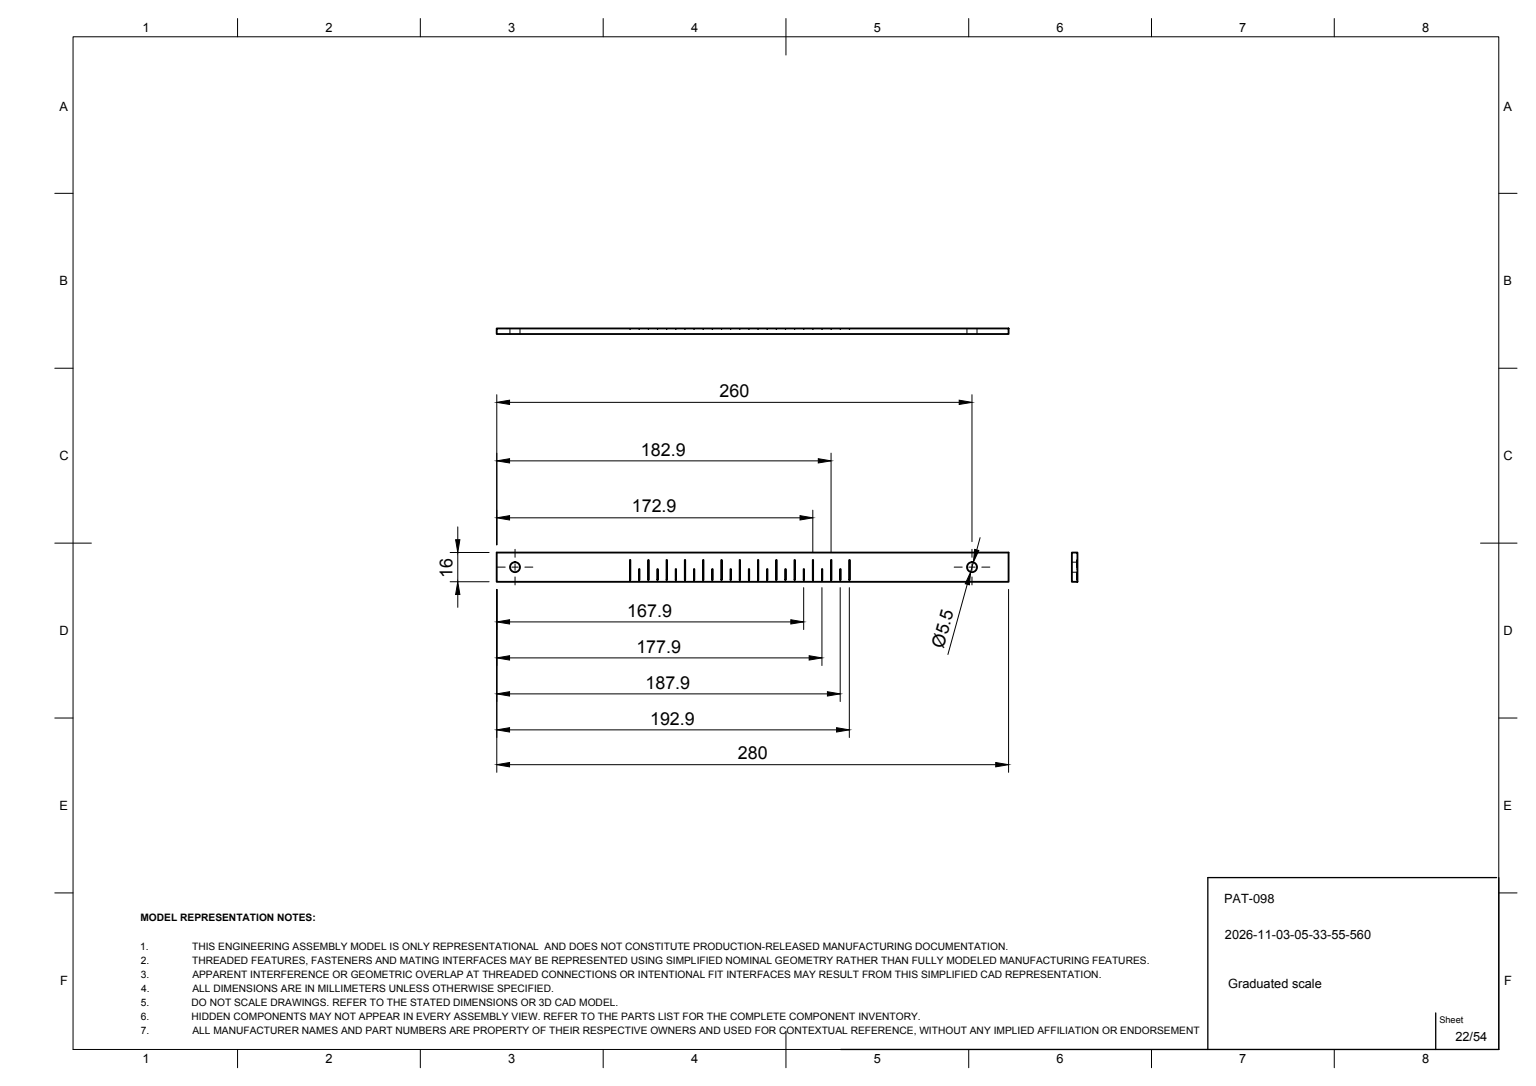
ISO-10303-21;
HEADER;
/* Generated by software containing ST-Developer
 * from STEP Tools, Inc. (www.steptools.com) 
 */

FILE_DESCRIPTION(
/* description */ ('Spring compression tester'),
/* implementation_level */ '2;1');

FILE_NAME(
/* name */ 'Graduated scale.step',
/* time_stamp */ '2026-10-28T03:24:11-07:00',
/* author */ (''),
/* organization */ (''),
/* preprocessor_version */ 'ST-DEVELOPER v20.2',
/* originating_system */ 'Autodesk Translation Framework v15.17.0.0',
/* authorisation */ '');

FILE_SCHEMA (('AUTOMOTIVE_DESIGN { 1 0 10303 214 3 1 1 }'));
ENDSEC;

DATA;
#10=MECHANICAL_DESIGN_GEOMETRIC_PRESENTATION_REPRESENTATION('',(#1123),#43521);
#1003=SHAPE_REPRESENTATION_RELATIONSHIP('SRR','None',#43815,#1063);
#1063=ADVANCED_BREP_SHAPE_REPRESENTATION('',(#1198),#43475);
#1123=STYLED_ITEM('',(#44216),#1198);
#1198=MANIFOLD_SOLID_BREP('Body1',#18560);
#1410=FACE_BOUND('',#3758,.T.);
#1411=FACE_BOUND('',#3759,.T.);
#1412=FACE_BOUND('',#3762,.T.);
#1413=FACE_BOUND('',#3763,.T.);
#1414=FACE_BOUND('',#3764,.T.);
#1415=FACE_BOUND('',#3765,.T.);
#1416=FACE_BOUND('',#3766,.T.);
#1417=FACE_BOUND('',#3767,.T.);
#1418=FACE_BOUND('',#3768,.T.);
#1419=FACE_BOUND('',#3769,.T.);
#1420=FACE_BOUND('',#3770,.T.);
#1421=FACE_BOUND('',#3771,.T.);
#1422=FACE_BOUND('',#3772,.T.);
#1423=FACE_BOUND('',#3773,.T.);
#1424=FACE_BOUND('',#3774,.T.);
#1425=FACE_BOUND('',#3775,.T.);
#1426=FACE_BOUND('',#3776,.T.);
#1427=FACE_BOUND('',#3777,.T.);
#1428=FACE_BOUND('',#3778,.T.);
#1429=FACE_BOUND('',#3779,.T.);
#1430=FACE_BOUND('',#3780,.T.);
#1431=FACE_BOUND('',#3781,.T.);
#1432=FACE_BOUND('',#3782,.T.);
#1433=FACE_BOUND('',#3783,.T.);
#1434=FACE_BOUND('',#3784,.T.);
#1435=FACE_BOUND('',#3785,.T.);
#1436=FACE_BOUND('',#3786,.T.);
#1437=FACE_BOUND('',#3787,.T.);
#1438=FACE_BOUND('',#3788,.T.);
#1728=PLANE('',#19783);
#1729=PLANE('',#19784);
#1730=PLANE('',#19785);
#1731=PLANE('',#19786);
#1732=PLANE('',#19787);
#1733=PLANE('',#19788);
#1734=PLANE('',#19789);
#1735=PLANE('',#19790);
#1736=PLANE('',#19791);
#1737=PLANE('',#19792);
#1738=PLANE('',#19793);
#1739=PLANE('',#19794);
#1740=PLANE('',#19795);
#1741=PLANE('',#19796);
#1742=PLANE('',#19797);
#1743=PLANE('',#19798);
#1744=PLANE('',#19799);
#1745=PLANE('',#19800);
#1746=PLANE('',#19801);
#1747=PLANE('',#19802);
#1748=PLANE('',#19803);
#1749=PLANE('',#19804);
#1750=PLANE('',#19805);
#1751=PLANE('',#19806);
#1752=PLANE('',#19807);
#1753=PLANE('',#19808);
#1754=PLANE('',#19809);
#1755=PLANE('',#19810);
#1756=PLANE('',#19811);
#1757=PLANE('',#19812);
#1758=PLANE('',#19813);
#1759=PLANE('',#19814);
#1760=PLANE('',#19815);
#1761=PLANE('',#19816);
#1762=PLANE('',#19817);
#1763=PLANE('',#19818);
#1764=PLANE('',#19819);
#1765=PLANE('',#19820);
#1766=PLANE('',#19821);
#1767=PLANE('',#19822);
#1768=PLANE('',#19823);
#1769=PLANE('',#19824);
#1770=PLANE('',#19825);
#1771=PLANE('',#19826);
#1772=PLANE('',#19827);
#1773=PLANE('',#19828);
#1774=PLANE('',#19829);
#1775=PLANE('',#19830);
#1776=PLANE('',#19831);
#1777=PLANE('',#19832);
#1778=PLANE('',#19833);
#1779=PLANE('',#19834);
#1780=PLANE('',#19835);
#1781=PLANE('',#19836);
#1782=PLANE('',#19837);
#1783=PLANE('',#19838);
#1784=PLANE('',#19839);
#1785=PLANE('',#19840);
#1786=PLANE('',#19841);
#1787=PLANE('',#19842);
#1788=PLANE('',#19843);
#1789=PLANE('',#19844);
#1790=PLANE('',#19845);
#1791=PLANE('',#19846);
#1792=PLANE('',#19847);
#1793=PLANE('',#19848);
#1794=PLANE('',#19849);
#1795=PLANE('',#19850);
#1796=PLANE('',#19851);
#1797=PLANE('',#19852);
#1798=PLANE('',#19853);
#1799=PLANE('',#19854);
#1800=PLANE('',#19855);
#1801=PLANE('',#19856);
#1802=PLANE('',#19857);
#1803=PLANE('',#19858);
#1804=PLANE('',#19859);
#1805=PLANE('',#19860);
#1806=PLANE('',#19861);
#1807=PLANE('',#19862);
#1808=PLANE('',#19863);
#1809=PLANE('',#19864);
#1810=PLANE('',#19865);
#1811=PLANE('',#19866);
#1812=PLANE('',#19867);
#1813=PLANE('',#19868);
#1814=PLANE('',#19869);
#1815=PLANE('',#19870);
#1816=PLANE('',#19871);
#1817=PLANE('',#19872);
#1818=PLANE('',#19873);
#1819=PLANE('',#19874);
#1820=PLANE('',#19875);
#1821=PLANE('',#19876);
#1822=PLANE('',#19877);
#1823=PLANE('',#19878);
#1824=PLANE('',#19879);
#1825=PLANE('',#19880);
#1826=PLANE('',#19881);
#1827=PLANE('',#19882);
#1828=PLANE('',#19883);
#1829=PLANE('',#19884);
#1830=PLANE('',#19885);
#1831=PLANE('',#19886);
#1832=PLANE('',#19887);
#1833=PLANE('',#19888);
#1834=PLANE('',#19889);
#1835=PLANE('',#19890);
#1836=PLANE('',#19891);
#1837=PLANE('',#19892);
#1838=PLANE('',#19893);
#1839=PLANE('',#19894);
#1840=PLANE('',#19895);
#1841=PLANE('',#19896);
#1842=PLANE('',#19897);
#1843=PLANE('',#19898);
#1844=PLANE('',#19899);
#1845=PLANE('',#19900);
#1846=PLANE('',#19901);
#1847=PLANE('',#19902);
#1848=PLANE('',#19903);
#1849=PLANE('',#19904);
#1850=PLANE('',#19905);
#1851=PLANE('',#19906);
#1852=PLANE('',#19907);
#1853=PLANE('',#19914);
#1854=PLANE('',#19915);
#1855=PLANE('',#19916);
#1856=PLANE('',#19917);
#1857=PLANE('',#19918);
#1858=PLANE('',#19919);
#2419=FACE_OUTER_BOUND('',#3629,.T.);
#2420=FACE_OUTER_BOUND('',#3630,.T.);
#2421=FACE_OUTER_BOUND('',#3631,.T.);
#2422=FACE_OUTER_BOUND('',#3632,.T.);
#2423=FACE_OUTER_BOUND('',#3633,.T.);
#2424=FACE_OUTER_BOUND('',#3634,.T.);
#2425=FACE_OUTER_BOUND('',#3635,.T.);
#2426=FACE_OUTER_BOUND('',#3636,.T.);
#2427=FACE_OUTER_BOUND('',#3637,.T.);
#2428=FACE_OUTER_BOUND('',#3638,.T.);
#2429=FACE_OUTER_BOUND('',#3639,.T.);
#2430=FACE_OUTER_BOUND('',#3640,.T.);
#2431=FACE_OUTER_BOUND('',#3641,.T.);
#2432=FACE_OUTER_BOUND('',#3642,.T.);
#2433=FACE_OUTER_BOUND('',#3643,.T.);
#2434=FACE_OUTER_BOUND('',#3644,.T.);
#2435=FACE_OUTER_BOUND('',#3645,.T.);
#2436=FACE_OUTER_BOUND('',#3646,.T.);
#2437=FACE_OUTER_BOUND('',#3647,.T.);
#2438=FACE_OUTER_BOUND('',#3648,.T.);
#2439=FACE_OUTER_BOUND('',#3649,.T.);
#2440=FACE_OUTER_BOUND('',#3650,.T.);
#2441=FACE_OUTER_BOUND('',#3651,.T.);
#2442=FACE_OUTER_BOUND('',#3652,.T.);
#2443=FACE_OUTER_BOUND('',#3653,.T.);
#2444=FACE_OUTER_BOUND('',#3654,.T.);
#2445=FACE_OUTER_BOUND('',#3655,.T.);
#2446=FACE_OUTER_BOUND('',#3656,.T.);
#2447=FACE_OUTER_BOUND('',#3657,.T.);
#2448=FACE_OUTER_BOUND('',#3658,.T.);
#2449=FACE_OUTER_BOUND('',#3659,.T.);
#2450=FACE_OUTER_BOUND('',#3660,.T.);
#2451=FACE_OUTER_BOUND('',#3661,.T.);
#2452=FACE_OUTER_BOUND('',#3662,.T.);
#2453=FACE_OUTER_BOUND('',#3663,.T.);
#2454=FACE_OUTER_BOUND('',#3664,.T.);
#2455=FACE_OUTER_BOUND('',#3665,.T.);
#2456=FACE_OUTER_BOUND('',#3666,.T.);
#2457=FACE_OUTER_BOUND('',#3667,.T.);
#2458=FACE_OUTER_BOUND('',#3668,.T.);
#2459=FACE_OUTER_BOUND('',#3669,.T.);
#2460=FACE_OUTER_BOUND('',#3670,.T.);
#2461=FACE_OUTER_BOUND('',#3671,.T.);
#2462=FACE_OUTER_BOUND('',#3672,.T.);
#2463=FACE_OUTER_BOUND('',#3673,.T.);
#2464=FACE_OUTER_BOUND('',#3674,.T.);
#2465=FACE_OUTER_BOUND('',#3675,.T.);
#2466=FACE_OUTER_BOUND('',#3676,.T.);
#2467=FACE_OUTER_BOUND('',#3677,.T.);
#2468=FACE_OUTER_BOUND('',#3678,.T.);
#2469=FACE_OUTER_BOUND('',#3679,.T.);
#2470=FACE_OUTER_BOUND('',#3680,.T.);
#2471=FACE_OUTER_BOUND('',#3681,.T.);
#2472=FACE_OUTER_BOUND('',#3682,.T.);
#2473=FACE_OUTER_BOUND('',#3683,.T.);
#2474=FACE_OUTER_BOUND('',#3684,.T.);
#2475=FACE_OUTER_BOUND('',#3685,.T.);
#2476=FACE_OUTER_BOUND('',#3686,.T.);
#2477=FACE_OUTER_BOUND('',#3687,.T.);
#2478=FACE_OUTER_BOUND('',#3688,.T.);
#2479=FACE_OUTER_BOUND('',#3689,.T.);
#2480=FACE_OUTER_BOUND('',#3690,.T.);
#2481=FACE_OUTER_BOUND('',#3691,.T.);
#2482=FACE_OUTER_BOUND('',#3692,.T.);
#2483=FACE_OUTER_BOUND('',#3693,.T.);
#2484=FACE_OUTER_BOUND('',#3694,.T.);
#2485=FACE_OUTER_BOUND('',#3695,.T.);
#2486=FACE_OUTER_BOUND('',#3696,.T.);
#2487=FACE_OUTER_BOUND('',#3697,.T.);
#2488=FACE_OUTER_BOUND('',#3698,.T.);
#2489=FACE_OUTER_BOUND('',#3699,.T.);
#2490=FACE_OUTER_BOUND('',#3700,.T.);
#2491=FACE_OUTER_BOUND('',#3701,.T.);
#2492=FACE_OUTER_BOUND('',#3702,.T.);
#2493=FACE_OUTER_BOUND('',#3703,.T.);
#2494=FACE_OUTER_BOUND('',#3704,.T.);
#2495=FACE_OUTER_BOUND('',#3705,.T.);
#2496=FACE_OUTER_BOUND('',#3706,.T.);
#2497=FACE_OUTER_BOUND('',#3707,.T.);
#2498=FACE_OUTER_BOUND('',#3708,.T.);
#2499=FACE_OUTER_BOUND('',#3709,.T.);
#2500=FACE_OUTER_BOUND('',#3710,.T.);
#2501=FACE_OUTER_BOUND('',#3711,.T.);
#2502=FACE_OUTER_BOUND('',#3712,.T.);
#2503=FACE_OUTER_BOUND('',#3713,.T.);
#2504=FACE_OUTER_BOUND('',#3714,.T.);
#2505=FACE_OUTER_BOUND('',#3715,.T.);
#2506=FACE_OUTER_BOUND('',#3716,.T.);
#2507=FACE_OUTER_BOUND('',#3717,.T.);
#2508=FACE_OUTER_BOUND('',#3718,.T.);
#2509=FACE_OUTER_BOUND('',#3719,.T.);
#2510=FACE_OUTER_BOUND('',#3720,.T.);
#2511=FACE_OUTER_BOUND('',#3721,.T.);
#2512=FACE_OUTER_BOUND('',#3722,.T.);
#2513=FACE_OUTER_BOUND('',#3723,.T.);
#2514=FACE_OUTER_BOUND('',#3724,.T.);
#2515=FACE_OUTER_BOUND('',#3725,.T.);
#2516=FACE_OUTER_BOUND('',#3726,.T.);
#2517=FACE_OUTER_BOUND('',#3727,.T.);
#2518=FACE_OUTER_BOUND('',#3728,.T.);
#2519=FACE_OUTER_BOUND('',#3729,.T.);
#2520=FACE_OUTER_BOUND('',#3730,.T.);
#2521=FACE_OUTER_BOUND('',#3731,.T.);
#2522=FACE_OUTER_BOUND('',#3732,.T.);
#2523=FACE_OUTER_BOUND('',#3733,.T.);
#2524=FACE_OUTER_BOUND('',#3734,.T.);
#2525=FACE_OUTER_BOUND('',#3735,.T.);
#2526=FACE_OUTER_BOUND('',#3736,.T.);
#2527=FACE_OUTER_BOUND('',#3737,.T.);
#2528=FACE_OUTER_BOUND('',#3738,.T.);
#2529=FACE_OUTER_BOUND('',#3739,.T.);
#2530=FACE_OUTER_BOUND('',#3740,.T.);
#2531=FACE_OUTER_BOUND('',#3741,.T.);
#2532=FACE_OUTER_BOUND('',#3742,.T.);
#2533=FACE_OUTER_BOUND('',#3743,.T.);
#2534=FACE_OUTER_BOUND('',#3744,.T.);
#2535=FACE_OUTER_BOUND('',#3745,.T.);
#2536=FACE_OUTER_BOUND('',#3746,.T.);
#2537=FACE_OUTER_BOUND('',#3747,.T.);
#2538=FACE_OUTER_BOUND('',#3748,.T.);
#2539=FACE_OUTER_BOUND('',#3749,.T.);
#2540=FACE_OUTER_BOUND('',#3750,.T.);
#2541=FACE_OUTER_BOUND('',#3751,.T.);
#2542=FACE_OUTER_BOUND('',#3752,.T.);
#2543=FACE_OUTER_BOUND('',#3753,.T.);
#2544=FACE_OUTER_BOUND('',#3754,.T.);
#2545=FACE_OUTER_BOUND('',#3755,.T.);
#2546=FACE_OUTER_BOUND('',#3756,.T.);
#2547=FACE_OUTER_BOUND('',#3757,.T.);
#2548=FACE_OUTER_BOUND('',#3760,.T.);
#2549=FACE_OUTER_BOUND('',#3761,.T.);
#2550=FACE_OUTER_BOUND('',#3789,.T.);
#2551=FACE_OUTER_BOUND('',#3790,.T.);
#3629=EDGE_LOOP('',(#13285,#13286,#13287,#13288));
#3630=EDGE_LOOP('',(#13289,#13290,#13291,#13292));
#3631=EDGE_LOOP('',(#13293,#13294,#13295,#13296));
#3632=EDGE_LOOP('',(#13297,#13298,#13299,#13300));
#3633=EDGE_LOOP('',(#13301,#13302,#13303,#13304));
#3634=EDGE_LOOP('',(#13305,#13306,#13307,#13308));
#3635=EDGE_LOOP('',(#13309,#13310,#13311,#13312));
#3636=EDGE_LOOP('',(#13313,#13314,#13315,#13316));
#3637=EDGE_LOOP('',(#13317,#13318,#13319,#13320));
#3638=EDGE_LOOP('',(#13321,#13322,#13323,#13324));
#3639=EDGE_LOOP('',(#13325,#13326,#13327,#13328));
#3640=EDGE_LOOP('',(#13329,#13330,#13331,#13332));
#3641=EDGE_LOOP('',(#13333,#13334,#13335,#13336));
#3642=EDGE_LOOP('',(#13337,#13338,#13339,#13340));
#3643=EDGE_LOOP('',(#13341,#13342,#13343,#13344));
#3644=EDGE_LOOP('',(#13345,#13346,#13347,#13348));
#3645=EDGE_LOOP('',(#13349,#13350,#13351,#13352));
#3646=EDGE_LOOP('',(#13353,#13354,#13355,#13356));
#3647=EDGE_LOOP('',(#13357,#13358,#13359,#13360));
#3648=EDGE_LOOP('',(#13361,#13362,#13363,#13364));
#3649=EDGE_LOOP('',(#13365,#13366,#13367,#13368));
#3650=EDGE_LOOP('',(#13369,#13370,#13371,#13372));
#3651=EDGE_LOOP('',(#13373,#13374,#13375,#13376));
#3652=EDGE_LOOP('',(#13377,#13378,#13379,#13380));
#3653=EDGE_LOOP('',(#13381,#13382,#13383,#13384));
#3654=EDGE_LOOP('',(#13385,#13386,#13387,#13388));
#3655=EDGE_LOOP('',(#13389,#13390,#13391,#13392));
#3656=EDGE_LOOP('',(#13393,#13394,#13395,#13396));
#3657=EDGE_LOOP('',(#13397,#13398,#13399,#13400));
#3658=EDGE_LOOP('',(#13401,#13402,#13403,#13404));
#3659=EDGE_LOOP('',(#13405,#13406,#13407,#13408));
#3660=EDGE_LOOP('',(#13409,#13410,#13411,#13412));
#3661=EDGE_LOOP('',(#13413,#13414,#13415,#13416));
#3662=EDGE_LOOP('',(#13417,#13418,#13419,#13420));
#3663=EDGE_LOOP('',(#13421,#13422,#13423,#13424));
#3664=EDGE_LOOP('',(#13425,#13426,#13427,#13428));
#3665=EDGE_LOOP('',(#13429,#13430,#13431,#13432));
#3666=EDGE_LOOP('',(#13433,#13434,#13435,#13436));
#3667=EDGE_LOOP('',(#13437,#13438,#13439,#13440));
#3668=EDGE_LOOP('',(#13441,#13442,#13443,#13444));
#3669=EDGE_LOOP('',(#13445,#13446,#13447,#13448));
#3670=EDGE_LOOP('',(#13449,#13450,#13451,#13452));
#3671=EDGE_LOOP('',(#13453,#13454,#13455,#13456));
#3672=EDGE_LOOP('',(#13457,#13458,#13459,#13460));
#3673=EDGE_LOOP('',(#13461,#13462,#13463,#13464));
#3674=EDGE_LOOP('',(#13465,#13466,#13467,#13468));
#3675=EDGE_LOOP('',(#13469,#13470,#13471,#13472));
#3676=EDGE_LOOP('',(#13473,#13474,#13475,#13476));
#3677=EDGE_LOOP('',(#13477,#13478,#13479,#13480));
#3678=EDGE_LOOP('',(#13481,#13482,#13483,#13484));
#3679=EDGE_LOOP('',(#13485,#13486,#13487,#13488));
#3680=EDGE_LOOP('',(#13489,#13490,#13491,#13492));
#3681=EDGE_LOOP('',(#13493,#13494,#13495,#13496));
#3682=EDGE_LOOP('',(#13497,#13498,#13499,#13500));
#3683=EDGE_LOOP('',(#13501,#13502,#13503,#13504));
#3684=EDGE_LOOP('',(#13505,#13506,#13507,#13508));
#3685=EDGE_LOOP('',(#13509,#13510,#13511,#13512));
#3686=EDGE_LOOP('',(#13513,#13514,#13515,#13516));
#3687=EDGE_LOOP('',(#13517,#13518,#13519,#13520));
#3688=EDGE_LOOP('',(#13521,#13522,#13523,#13524));
#3689=EDGE_LOOP('',(#13525,#13526,#13527,#13528));
#3690=EDGE_LOOP('',(#13529,#13530,#13531,#13532));
#3691=EDGE_LOOP('',(#13533,#13534,#13535,#13536));
#3692=EDGE_LOOP('',(#13537,#13538,#13539,#13540));
#3693=EDGE_LOOP('',(#13541,#13542,#13543,#13544));
#3694=EDGE_LOOP('',(#13545,#13546,#13547,#13548));
#3695=EDGE_LOOP('',(#13549,#13550,#13551,#13552));
#3696=EDGE_LOOP('',(#13553,#13554,#13555,#13556));
#3697=EDGE_LOOP('',(#13557,#13558,#13559,#13560));
#3698=EDGE_LOOP('',(#13561,#13562,#13563,#13564));
#3699=EDGE_LOOP('',(#13565,#13566,#13567,#13568));
#3700=EDGE_LOOP('',(#13569,#13570,#13571,#13572));
#3701=EDGE_LOOP('',(#13573,#13574,#13575,#13576));
#3702=EDGE_LOOP('',(#13577,#13578,#13579,#13580));
#3703=EDGE_LOOP('',(#13581,#13582,#13583,#13584));
#3704=EDGE_LOOP('',(#13585,#13586,#13587,#13588));
#3705=EDGE_LOOP('',(#13589,#13590,#13591,#13592));
#3706=EDGE_LOOP('',(#13593,#13594,#13595,#13596));
#3707=EDGE_LOOP('',(#13597,#13598,#13599,#13600));
#3708=EDGE_LOOP('',(#13601,#13602,#13603,#13604));
#3709=EDGE_LOOP('',(#13605,#13606,#13607,#13608));
#3710=EDGE_LOOP('',(#13609,#13610,#13611,#13612));
#3711=EDGE_LOOP('',(#13613,#13614,#13615,#13616));
#3712=EDGE_LOOP('',(#13617,#13618,#13619,#13620));
#3713=EDGE_LOOP('',(#13621,#13622,#13623,#13624));
#3714=EDGE_LOOP('',(#13625,#13626,#13627,#13628));
#3715=EDGE_LOOP('',(#13629,#13630,#13631,#13632));
#3716=EDGE_LOOP('',(#13633,#13634,#13635,#13636));
#3717=EDGE_LOOP('',(#13637,#13638,#13639,#13640));
#3718=EDGE_LOOP('',(#13641,#13642,#13643,#13644));
#3719=EDGE_LOOP('',(#13645,#13646,#13647,#13648));
#3720=EDGE_LOOP('',(#13649,#13650,#13651,#13652));
#3721=EDGE_LOOP('',(#13653,#13654,#13655,#13656));
#3722=EDGE_LOOP('',(#13657,#13658,#13659,#13660));
#3723=EDGE_LOOP('',(#13661,#13662,#13663,#13664));
#3724=EDGE_LOOP('',(#13665,#13666,#13667,#13668));
#3725=EDGE_LOOP('',(#13669,#13670,#13671,#13672));
#3726=EDGE_LOOP('',(#13673,#13674,#13675,#13676));
#3727=EDGE_LOOP('',(#13677,#13678,#13679,#13680));
#3728=EDGE_LOOP('',(#13681,#13682,#13683,#13684));
#3729=EDGE_LOOP('',(#13685,#13686,#13687,#13688));
#3730=EDGE_LOOP('',(#13689,#13690,#13691,#13692));
#3731=EDGE_LOOP('',(#13693,#13694,#13695,#13696));
#3732=EDGE_LOOP('',(#13697,#13698,#13699,#13700));
#3733=EDGE_LOOP('',(#13701,#13702,#13703,#13704));
#3734=EDGE_LOOP('',(#13705,#13706,#13707,#13708));
#3735=EDGE_LOOP('',(#13709,#13710,#13711,#13712));
#3736=EDGE_LOOP('',(#13713,#13714,#13715,#13716));
#3737=EDGE_LOOP('',(#13717,#13718,#13719,#13720));
#3738=EDGE_LOOP('',(#13721,#13722,#13723,#13724));
#3739=EDGE_LOOP('',(#13725,#13726,#13727,#13728));
#3740=EDGE_LOOP('',(#13729,#13730,#13731,#13732));
#3741=EDGE_LOOP('',(#13733,#13734,#13735,#13736));
#3742=EDGE_LOOP('',(#13737,#13738,#13739,#13740));
#3743=EDGE_LOOP('',(#13741,#13742,#13743,#13744));
#3744=EDGE_LOOP('',(#13745,#13746,#13747,#13748));
#3745=EDGE_LOOP('',(#13749,#13750,#13751,#13752));
#3746=EDGE_LOOP('',(#13753,#13754,#13755,#13756));
#3747=EDGE_LOOP('',(#13757,#13758,#13759,#13760));
#3748=EDGE_LOOP('',(#13761,#13762,#13763,#13764));
#3749=EDGE_LOOP('',(#13765,#13766,#13767,#13768));
#3750=EDGE_LOOP('',(#13769,#13770,#13771,#13772));
#3751=EDGE_LOOP('',(#13773,#13774,#13775,#13776));
#3752=EDGE_LOOP('',(#13777,#13778,#13779,#13780));
#3753=EDGE_LOOP('',(#13781,#13782,#13783,#13784));
#3754=EDGE_LOOP('',(#13785,#13786,#13787,#13788));
#3755=EDGE_LOOP('',(#13789,#13790,#13791,#13792));
#3756=EDGE_LOOP('',(#13793,#13794,#13795,#13796));
#3757=EDGE_LOOP('',(#13797,#13798,#13799,#13800));
#3758=EDGE_LOOP('',(#13801));
#3759=EDGE_LOOP('',(#13802));
#3760=EDGE_LOOP('',(#13803,#13804,#13805,#13806));
#3761=EDGE_LOOP('',(#13807,#13808,#13809,#13810));
#3762=EDGE_LOOP('',(#13811,#13812,#13813,#13814));
#3763=EDGE_LOOP('',(#13815,#13816,#13817,#13818));
#3764=EDGE_LOOP('',(#13819,#13820,#13821,#13822));
#3765=EDGE_LOOP('',(#13823,#13824,#13825,#13826));
#3766=EDGE_LOOP('',(#13827,#13828,#13829,#13830));
#3767=EDGE_LOOP('',(#13831,#13832,#13833,#13834));
#3768=EDGE_LOOP('',(#13835,#13836,#13837,#13838));
#3769=EDGE_LOOP('',(#13839,#13840,#13841,#13842));
#3770=EDGE_LOOP('',(#13843,#13844,#13845,#13846));
#3771=EDGE_LOOP('',(#13847,#13848,#13849,#13850));
#3772=EDGE_LOOP('',(#13851,#13852,#13853,#13854));
#3773=EDGE_LOOP('',(#13855,#13856,#13857,#13858));
#3774=EDGE_LOOP('',(#13859,#13860,#13861,#13862));
#3775=EDGE_LOOP('',(#13863,#13864,#13865,#13866));
#3776=EDGE_LOOP('',(#13867,#13868,#13869,#13870));
#3777=EDGE_LOOP('',(#13871));
#3778=EDGE_LOOP('',(#13872));
#3779=EDGE_LOOP('',(#13873,#13874,#13875,#13876));
#3780=EDGE_LOOP('',(#13877,#13878,#13879,#13880));
#3781=EDGE_LOOP('',(#13881,#13882,#13883,#13884));
#3782=EDGE_LOOP('',(#13885,#13886,#13887,#13888));
#3783=EDGE_LOOP('',(#13889,#13890,#13891,#13892));
#3784=EDGE_LOOP('',(#13893,#13894,#13895,#13896));
#3785=EDGE_LOOP('',(#13897,#13898,#13899,#13900));
#3786=EDGE_LOOP('',(#13901,#13902,#13903,#13904));
#3787=EDGE_LOOP('',(#13905,#13906,#13907,#13908));
#3788=EDGE_LOOP('',(#13909,#13910,#13911,#13912));
#3789=EDGE_LOOP('',(#13913,#13914,#13915,#13916));
#3790=EDGE_LOOP('',(#13917,#13918,#13919,#13920));
#4912=LINE('',#27616,#6344);
#4913=LINE('',#27618,#6345);
#4914=LINE('',#27620,#6346);
#4915=LINE('',#27621,#6347);
#4916=LINE('',#27624,#6348);
#4917=LINE('',#27626,#6349);
#4918=LINE('',#27627,#6350);
#4919=LINE('',#27630,#6351);
#4920=LINE('',#27632,#6352);
#4921=LINE('',#27633,#6353);
#4922=LINE('',#27635,#6354);
#4923=LINE('',#27636,#6355);
#4924=LINE('',#27641,#6356);
#4925=LINE('',#27643,#6357);
#4926=LINE('',#27645,#6358);
#4927=LINE('',#27646,#6359);
#4928=LINE('',#27649,#6360);
#4929=LINE('',#27651,#6361);
#4930=LINE('',#27652,#6362);
#4931=LINE('',#27655,#6363);
#4932=LINE('',#27657,#6364);
#4933=LINE('',#27658,#6365);
#4934=LINE('',#27660,#6366);
#4935=LINE('',#27661,#6367);
#4936=LINE('',#27666,#6368);
#4937=LINE('',#27668,#6369);
#4938=LINE('',#27670,#6370);
#4939=LINE('',#27671,#6371);
#4940=LINE('',#27674,#6372);
#4941=LINE('',#27676,#6373);
#4942=LINE('',#27677,#6374);
#4943=LINE('',#27680,#6375);
#4944=LINE('',#27682,#6376);
#4945=LINE('',#27683,#6377);
#4946=LINE('',#27685,#6378);
#4947=LINE('',#27686,#6379);
#4948=LINE('',#27691,#6380);
#4949=LINE('',#27693,#6381);
#4950=LINE('',#27695,#6382);
#4951=LINE('',#27696,#6383);
#4952=LINE('',#27699,#6384);
#4953=LINE('',#27701,#6385);
#4954=LINE('',#27702,#6386);
#4955=LINE('',#27705,#6387);
#4956=LINE('',#27707,#6388);
#4957=LINE('',#27708,#6389);
#4958=LINE('',#27710,#6390);
#4959=LINE('',#27711,#6391);
#4960=LINE('',#27716,#6392);
#4961=LINE('',#27718,#6393);
#4962=LINE('',#27720,#6394);
#4963=LINE('',#27721,#6395);
#4964=LINE('',#27724,#6396);
#4965=LINE('',#27726,#6397);
#4966=LINE('',#27727,#6398);
#4967=LINE('',#27730,#6399);
#4968=LINE('',#27732,#6400);
#4969=LINE('',#27733,#6401);
#4970=LINE('',#27735,#6402);
#4971=LINE('',#27736,#6403);
#4972=LINE('',#27741,#6404);
#4973=LINE('',#27743,#6405);
#4974=LINE('',#27745,#6406);
#4975=LINE('',#27746,#6407);
#4976=LINE('',#27749,#6408);
#4977=LINE('',#27751,#6409);
#4978=LINE('',#27752,#6410);
#4979=LINE('',#27755,#6411);
#4980=LINE('',#27757,#6412);
#4981=LINE('',#27758,#6413);
#4982=LINE('',#27760,#6414);
#4983=LINE('',#27761,#6415);
#4984=LINE('',#27766,#6416);
#4985=LINE('',#27768,#6417);
#4986=LINE('',#27770,#6418);
#4987=LINE('',#27771,#6419);
#4988=LINE('',#27774,#6420);
#4989=LINE('',#27776,#6421);
#4990=LINE('',#27777,#6422);
#4991=LINE('',#27780,#6423);
#4992=LINE('',#27782,#6424);
#4993=LINE('',#27783,#6425);
#4994=LINE('',#27785,#6426);
#4995=LINE('',#27786,#6427);
#4996=LINE('',#27791,#6428);
#4997=LINE('',#27793,#6429);
#4998=LINE('',#27795,#6430);
#4999=LINE('',#27796,#6431);
#5000=LINE('',#27799,#6432);
#5001=LINE('',#27801,#6433);
#5002=LINE('',#27802,#6434);
#5003=LINE('',#27805,#6435);
#5004=LINE('',#27807,#6436);
#5005=LINE('',#27808,#6437);
#5006=LINE('',#27810,#6438);
#5007=LINE('',#27811,#6439);
#5008=LINE('',#27816,#6440);
#5009=LINE('',#27818,#6441);
#5010=LINE('',#27820,#6442);
#5011=LINE('',#27821,#6443);
#5012=LINE('',#27824,#6444);
#5013=LINE('',#27826,#6445);
#5014=LINE('',#27827,#6446);
#5015=LINE('',#27830,#6447);
#5016=LINE('',#27832,#6448);
#5017=LINE('',#27833,#6449);
#5018=LINE('',#27835,#6450);
#5019=LINE('',#27836,#6451);
#5020=LINE('',#27841,#6452);
#5021=LINE('',#27843,#6453);
#5022=LINE('',#27845,#6454);
#5023=LINE('',#27846,#6455);
#5024=LINE('',#27849,#6456);
#5025=LINE('',#27851,#6457);
#5026=LINE('',#27852,#6458);
#5027=LINE('',#27855,#6459);
#5028=LINE('',#27857,#6460);
#5029=LINE('',#27858,#6461);
#5030=LINE('',#27860,#6462);
#5031=LINE('',#27861,#6463);
#5032=LINE('',#27866,#6464);
#5033=LINE('',#27868,#6465);
#5034=LINE('',#27870,#6466);
#5035=LINE('',#27871,#6467);
#5036=LINE('',#27874,#6468);
#5037=LINE('',#27876,#6469);
#5038=LINE('',#27877,#6470);
#5039=LINE('',#27880,#6471);
#5040=LINE('',#27882,#6472);
#5041=LINE('',#27883,#6473);
#5042=LINE('',#27885,#6474);
#5043=LINE('',#27886,#6475);
#5044=LINE('',#27891,#6476);
#5045=LINE('',#27893,#6477);
#5046=LINE('',#27895,#6478);
#5047=LINE('',#27896,#6479);
#5048=LINE('',#27899,#6480);
#5049=LINE('',#27901,#6481);
#5050=LINE('',#27902,#6482);
#5051=LINE('',#27905,#6483);
#5052=LINE('',#27907,#6484);
#5053=LINE('',#27908,#6485);
#5054=LINE('',#27910,#6486);
#5055=LINE('',#27911,#6487);
#5056=LINE('',#27916,#6488);
#5057=LINE('',#27918,#6489);
#5058=LINE('',#27920,#6490);
#5059=LINE('',#27921,#6491);
#5060=LINE('',#27924,#6492);
#5061=LINE('',#27926,#6493);
#5062=LINE('',#27927,#6494);
#5063=LINE('',#27930,#6495);
#5064=LINE('',#27932,#6496);
#5065=LINE('',#27933,#6497);
#5066=LINE('',#27935,#6498);
#5067=LINE('',#27936,#6499);
#5068=LINE('',#27941,#6500);
#5069=LINE('',#27943,#6501);
#5070=LINE('',#27945,#6502);
#5071=LINE('',#27946,#6503);
#5072=LINE('',#27949,#6504);
#5073=LINE('',#27951,#6505);
#5074=LINE('',#27952,#6506);
#5075=LINE('',#27955,#6507);
#5076=LINE('',#27957,#6508);
#5077=LINE('',#27958,#6509);
#5078=LINE('',#27960,#6510);
#5079=LINE('',#27961,#6511);
#5080=LINE('',#27966,#6512);
#5081=LINE('',#27968,#6513);
#5082=LINE('',#27970,#6514);
#5083=LINE('',#27971,#6515);
#5084=LINE('',#27974,#6516);
#5085=LINE('',#27976,#6517);
#5086=LINE('',#27977,#6518);
#5087=LINE('',#27980,#6519);
#5088=LINE('',#27982,#6520);
#5089=LINE('',#27983,#6521);
#5090=LINE('',#27985,#6522);
#5091=LINE('',#27986,#6523);
#5092=LINE('',#27991,#6524);
#5093=LINE('',#27993,#6525);
#5094=LINE('',#27995,#6526);
#5095=LINE('',#27996,#6527);
#5096=LINE('',#27999,#6528);
#5097=LINE('',#28001,#6529);
#5098=LINE('',#28002,#6530);
#5099=LINE('',#28005,#6531);
#5100=LINE('',#28007,#6532);
#5101=LINE('',#28008,#6533);
#5102=LINE('',#28010,#6534);
#5103=LINE('',#28011,#6535);
#5104=LINE('',#28016,#6536);
#5105=LINE('',#28018,#6537);
#5106=LINE('',#28020,#6538);
#5107=LINE('',#28021,#6539);
#5108=LINE('',#28024,#6540);
#5109=LINE('',#28026,#6541);
#5110=LINE('',#28027,#6542);
#5111=LINE('',#28030,#6543);
#5112=LINE('',#28032,#6544);
#5113=LINE('',#28033,#6545);
#5114=LINE('',#28035,#6546);
#5115=LINE('',#28036,#6547);
#5116=LINE('',#28041,#6548);
#5117=LINE('',#28043,#6549);
#5118=LINE('',#28045,#6550);
#5119=LINE('',#28046,#6551);
#5120=LINE('',#28049,#6552);
#5121=LINE('',#28051,#6553);
#5122=LINE('',#28052,#6554);
#5123=LINE('',#28055,#6555);
#5124=LINE('',#28057,#6556);
#5125=LINE('',#28058,#6557);
#5126=LINE('',#28060,#6558);
#5127=LINE('',#28061,#6559);
#5128=LINE('',#28066,#6560);
#5129=LINE('',#28068,#6561);
#5130=LINE('',#28070,#6562);
#5131=LINE('',#28071,#6563);
#5132=LINE('',#28074,#6564);
#5133=LINE('',#28076,#6565);
#5134=LINE('',#28077,#6566);
#5135=LINE('',#28080,#6567);
#5136=LINE('',#28082,#6568);
#5137=LINE('',#28083,#6569);
#5138=LINE('',#28085,#6570);
#5139=LINE('',#28086,#6571);
#5140=LINE('',#28091,#6572);
#5141=LINE('',#28093,#6573);
#5142=LINE('',#28095,#6574);
#5143=LINE('',#28096,#6575);
#5144=LINE('',#28099,#6576);
#5145=LINE('',#28101,#6577);
#5146=LINE('',#28102,#6578);
#5147=LINE('',#28105,#6579);
#5148=LINE('',#28107,#6580);
#5149=LINE('',#28108,#6581);
#5150=LINE('',#28110,#6582);
#5151=LINE('',#28111,#6583);
#5152=LINE('',#28116,#6584);
#5153=LINE('',#28118,#6585);
#5154=LINE('',#28120,#6586);
#5155=LINE('',#28121,#6587);
#5156=LINE('',#28124,#6588);
#5157=LINE('',#28126,#6589);
#5158=LINE('',#28127,#6590);
#5159=LINE('',#28130,#6591);
#5160=LINE('',#28132,#6592);
#5161=LINE('',#28133,#6593);
#5162=LINE('',#28135,#6594);
#5163=LINE('',#28136,#6595);
#5164=LINE('',#28141,#6596);
#5165=LINE('',#28143,#6597);
#5166=LINE('',#28145,#6598);
#5167=LINE('',#28146,#6599);
#5168=LINE('',#28149,#6600);
#5169=LINE('',#28151,#6601);
#5170=LINE('',#28152,#6602);
#5171=LINE('',#28155,#6603);
#5172=LINE('',#28157,#6604);
#5173=LINE('',#28158,#6605);
#5174=LINE('',#28160,#6606);
#5175=LINE('',#28161,#6607);
#5176=LINE('',#28166,#6608);
#5177=LINE('',#28168,#6609);
#5178=LINE('',#28170,#6610);
#5179=LINE('',#28171,#6611);
#5180=LINE('',#28174,#6612);
#5181=LINE('',#28176,#6613);
#5182=LINE('',#28177,#6614);
#5183=LINE('',#28180,#6615);
#5184=LINE('',#28182,#6616);
#5185=LINE('',#28183,#6617);
#5186=LINE('',#28185,#6618);
#5187=LINE('',#28186,#6619);
#5188=LINE('',#28191,#6620);
#5189=LINE('',#28193,#6621);
#5190=LINE('',#28195,#6622);
#5191=LINE('',#28196,#6623);
#5192=LINE('',#28199,#6624);
#5193=LINE('',#28201,#6625);
#5194=LINE('',#28202,#6626);
#5195=LINE('',#28205,#6627);
#5196=LINE('',#28207,#6628);
#5197=LINE('',#28208,#6629);
#5198=LINE('',#28210,#6630);
#5199=LINE('',#28211,#6631);
#5200=LINE('',#28216,#6632);
#5201=LINE('',#28218,#6633);
#5202=LINE('',#28220,#6634);
#5203=LINE('',#28221,#6635);
#5204=LINE('',#28224,#6636);
#5205=LINE('',#28226,#6637);
#5206=LINE('',#28227,#6638);
#5207=LINE('',#28230,#6639);
#5208=LINE('',#28232,#6640);
#5209=LINE('',#28233,#6641);
#5210=LINE('',#28235,#6642);
#5211=LINE('',#28236,#6643);
#5212=LINE('',#28242,#6644);
#5213=LINE('',#28248,#6645);
#5214=LINE('',#28253,#6646);
#5215=LINE('',#28255,#6647);
#5216=LINE('',#28257,#6648);
#5217=LINE('',#28258,#6649);
#5218=LINE('',#28261,#6650);
#5219=LINE('',#28263,#6651);
#5220=LINE('',#28264,#6652);
#5221=LINE('',#28267,#6653);
#5222=LINE('',#28269,#6654);
#5223=LINE('',#28270,#6655);
#5224=LINE('',#28272,#6656);
#5225=LINE('',#28273,#6657);
#6344=VECTOR('',#22502,1.);
#6345=VECTOR('',#22503,1.);
#6346=VECTOR('',#22504,1.);
#6347=VECTOR('',#22505,1.);
#6348=VECTOR('',#22508,1.);
#6349=VECTOR('',#22509,1.);
#6350=VECTOR('',#22510,1.);
#6351=VECTOR('',#22513,1.);
#6352=VECTOR('',#22514,1.);
#6353=VECTOR('',#22515,1.);
#6354=VECTOR('',#22518,1.);
#6355=VECTOR('',#22519,1.);
#6356=VECTOR('',#22524,1.);
#6357=VECTOR('',#22525,1.);
#6358=VECTOR('',#22526,1.);
#6359=VECTOR('',#22527,1.);
#6360=VECTOR('',#22530,1.);
#6361=VECTOR('',#22531,1.);
#6362=VECTOR('',#22532,1.);
#6363=VECTOR('',#22535,1.);
#6364=VECTOR('',#22536,1.);
#6365=VECTOR('',#22537,1.);
#6366=VECTOR('',#22540,1.);
#6367=VECTOR('',#22541,1.);
#6368=VECTOR('',#22546,1.);
#6369=VECTOR('',#22547,1.);
#6370=VECTOR('',#22548,1.);
#6371=VECTOR('',#22549,1.);
#6372=VECTOR('',#22552,1.);
#6373=VECTOR('',#22553,1.);
#6374=VECTOR('',#22554,1.);
#6375=VECTOR('',#22557,1.);
#6376=VECTOR('',#22558,1.);
#6377=VECTOR('',#22559,1.);
#6378=VECTOR('',#22562,1.);
#6379=VECTOR('',#22563,1.);
#6380=VECTOR('',#22568,1.);
#6381=VECTOR('',#22569,1.);
#6382=VECTOR('',#22570,1.);
#6383=VECTOR('',#22571,1.);
#6384=VECTOR('',#22574,1.);
#6385=VECTOR('',#22575,1.);
#6386=VECTOR('',#22576,1.);
#6387=VECTOR('',#22579,1.);
#6388=VECTOR('',#22580,1.);
#6389=VECTOR('',#22581,1.);
#6390=VECTOR('',#22584,1.);
#6391=VECTOR('',#22585,1.);
#6392=VECTOR('',#22590,1.);
#6393=VECTOR('',#22591,1.);
#6394=VECTOR('',#22592,1.);
#6395=VECTOR('',#22593,1.);
#6396=VECTOR('',#22596,1.);
#6397=VECTOR('',#22597,1.);
#6398=VECTOR('',#22598,1.);
#6399=VECTOR('',#22601,1.);
#6400=VECTOR('',#22602,1.);
#6401=VECTOR('',#22603,1.);
#6402=VECTOR('',#22606,1.);
#6403=VECTOR('',#22607,1.);
#6404=VECTOR('',#22612,1.);
#6405=VECTOR('',#22613,1.);
#6406=VECTOR('',#22614,1.);
#6407=VECTOR('',#22615,1.);
#6408=VECTOR('',#22618,1.);
#6409=VECTOR('',#22619,1.);
#6410=VECTOR('',#22620,1.);
#6411=VECTOR('',#22623,1.);
#6412=VECTOR('',#22624,1.);
#6413=VECTOR('',#22625,1.);
#6414=VECTOR('',#22628,1.);
#6415=VECTOR('',#22629,1.);
#6416=VECTOR('',#22634,1.);
#6417=VECTOR('',#22635,1.);
#6418=VECTOR('',#22636,1.);
#6419=VECTOR('',#22637,1.);
#6420=VECTOR('',#22640,1.);
#6421=VECTOR('',#22641,1.);
#6422=VECTOR('',#22642,1.);
#6423=VECTOR('',#22645,1.);
#6424=VECTOR('',#22646,1.);
#6425=VECTOR('',#22647,1.);
#6426=VECTOR('',#22650,1.);
#6427=VECTOR('',#22651,1.);
#6428=VECTOR('',#22656,1.);
#6429=VECTOR('',#22657,1.);
#6430=VECTOR('',#22658,1.);
#6431=VECTOR('',#22659,1.);
#6432=VECTOR('',#22662,1.);
#6433=VECTOR('',#22663,1.);
#6434=VECTOR('',#22664,1.);
#6435=VECTOR('',#22667,1.);
#6436=VECTOR('',#22668,1.);
#6437=VECTOR('',#22669,1.);
#6438=VECTOR('',#22672,1.);
#6439=VECTOR('',#22673,1.);
#6440=VECTOR('',#22678,1.);
#6441=VECTOR('',#22679,1.);
#6442=VECTOR('',#22680,1.);
#6443=VECTOR('',#22681,1.);
#6444=VECTOR('',#22684,1.);
#6445=VECTOR('',#22685,1.);
#6446=VECTOR('',#22686,1.);
#6447=VECTOR('',#22689,1.);
#6448=VECTOR('',#22690,1.);
#6449=VECTOR('',#22691,1.);
#6450=VECTOR('',#22694,1.);
#6451=VECTOR('',#22695,1.);
#6452=VECTOR('',#22700,1.);
#6453=VECTOR('',#22701,1.);
#6454=VECTOR('',#22702,1.);
#6455=VECTOR('',#22703,1.);
#6456=VECTOR('',#22706,1.);
#6457=VECTOR('',#22707,1.);
#6458=VECTOR('',#22708,1.);
#6459=VECTOR('',#22711,1.);
#6460=VECTOR('',#22712,1.);
#6461=VECTOR('',#22713,1.);
#6462=VECTOR('',#22716,1.);
#6463=VECTOR('',#22717,1.);
#6464=VECTOR('',#22722,1.);
#6465=VECTOR('',#22723,1.);
#6466=VECTOR('',#22724,1.);
#6467=VECTOR('',#22725,1.);
#6468=VECTOR('',#22728,1.);
#6469=VECTOR('',#22729,1.);
#6470=VECTOR('',#22730,1.);
#6471=VECTOR('',#22733,1.);
#6472=VECTOR('',#22734,1.);
#6473=VECTOR('',#22735,1.);
#6474=VECTOR('',#22738,1.);
#6475=VECTOR('',#22739,1.);
#6476=VECTOR('',#22744,1.);
#6477=VECTOR('',#22745,1.);
#6478=VECTOR('',#22746,1.);
#6479=VECTOR('',#22747,1.);
#6480=VECTOR('',#22750,1.);
#6481=VECTOR('',#22751,1.);
#6482=VECTOR('',#22752,1.);
#6483=VECTOR('',#22755,1.);
#6484=VECTOR('',#22756,1.);
#6485=VECTOR('',#22757,1.);
#6486=VECTOR('',#22760,1.);
#6487=VECTOR('',#22761,1.);
#6488=VECTOR('',#22766,1.);
#6489=VECTOR('',#22767,1.);
#6490=VECTOR('',#22768,1.);
#6491=VECTOR('',#22769,1.);
#6492=VECTOR('',#22772,1.);
#6493=VECTOR('',#22773,1.);
#6494=VECTOR('',#22774,1.);
#6495=VECTOR('',#22777,1.);
#6496=VECTOR('',#22778,1.);
#6497=VECTOR('',#22779,1.);
#6498=VECTOR('',#22782,1.);
#6499=VECTOR('',#22783,1.);
#6500=VECTOR('',#22788,1.);
#6501=VECTOR('',#22789,1.);
#6502=VECTOR('',#22790,1.);
#6503=VECTOR('',#22791,1.);
#6504=VECTOR('',#22794,1.);
#6505=VECTOR('',#22795,1.);
#6506=VECTOR('',#22796,1.);
#6507=VECTOR('',#22799,1.);
#6508=VECTOR('',#22800,1.);
#6509=VECTOR('',#22801,1.);
#6510=VECTOR('',#22804,1.);
#6511=VECTOR('',#22805,1.);
#6512=VECTOR('',#22810,1.);
#6513=VECTOR('',#22811,1.);
#6514=VECTOR('',#22812,1.);
#6515=VECTOR('',#22813,1.);
#6516=VECTOR('',#22816,1.);
#6517=VECTOR('',#22817,1.);
#6518=VECTOR('',#22818,1.);
#6519=VECTOR('',#22821,1.);
#6520=VECTOR('',#22822,1.);
#6521=VECTOR('',#22823,1.);
#6522=VECTOR('',#22826,1.);
#6523=VECTOR('',#22827,1.);
#6524=VECTOR('',#22832,1.);
#6525=VECTOR('',#22833,1.);
#6526=VECTOR('',#22834,1.);
#6527=VECTOR('',#22835,1.);
#6528=VECTOR('',#22838,1.);
#6529=VECTOR('',#22839,1.);
#6530=VECTOR('',#22840,1.);
#6531=VECTOR('',#22843,1.);
#6532=VECTOR('',#22844,1.);
#6533=VECTOR('',#22845,1.);
#6534=VECTOR('',#22848,1.);
#6535=VECTOR('',#22849,1.);
#6536=VECTOR('',#22854,1.);
#6537=VECTOR('',#22855,1.);
#6538=VECTOR('',#22856,1.);
#6539=VECTOR('',#22857,1.);
#6540=VECTOR('',#22860,1.);
#6541=VECTOR('',#22861,1.);
#6542=VECTOR('',#22862,1.);
#6543=VECTOR('',#22865,1.);
#6544=VECTOR('',#22866,1.);
#6545=VECTOR('',#22867,1.);
#6546=VECTOR('',#22870,1.);
#6547=VECTOR('',#22871,1.);
#6548=VECTOR('',#22876,1.);
#6549=VECTOR('',#22877,1.);
#6550=VECTOR('',#22878,1.);
#6551=VECTOR('',#22879,1.);
#6552=VECTOR('',#22882,1.);
#6553=VECTOR('',#22883,1.);
#6554=VECTOR('',#22884,1.);
#6555=VECTOR('',#22887,1.);
#6556=VECTOR('',#22888,1.);
#6557=VECTOR('',#22889,1.);
#6558=VECTOR('',#22892,1.);
#6559=VECTOR('',#22893,1.);
#6560=VECTOR('',#22898,1.);
#6561=VECTOR('',#22899,1.);
#6562=VECTOR('',#22900,1.);
#6563=VECTOR('',#22901,1.);
#6564=VECTOR('',#22904,1.);
#6565=VECTOR('',#22905,1.);
#6566=VECTOR('',#22906,1.);
#6567=VECTOR('',#22909,1.);
#6568=VECTOR('',#22910,1.);
#6569=VECTOR('',#22911,1.);
#6570=VECTOR('',#22914,1.);
#6571=VECTOR('',#22915,1.);
#6572=VECTOR('',#22920,1.);
#6573=VECTOR('',#22921,1.);
#6574=VECTOR('',#22922,1.);
#6575=VECTOR('',#22923,1.);
#6576=VECTOR('',#22926,1.);
#6577=VECTOR('',#22927,1.);
#6578=VECTOR('',#22928,1.);
#6579=VECTOR('',#22931,1.);
#6580=VECTOR('',#22932,1.);
#6581=VECTOR('',#22933,1.);
#6582=VECTOR('',#22936,1.);
#6583=VECTOR('',#22937,1.);
#6584=VECTOR('',#22942,1.);
#6585=VECTOR('',#22943,1.);
#6586=VECTOR('',#22944,1.);
#6587=VECTOR('',#22945,1.);
#6588=VECTOR('',#22948,1.);
#6589=VECTOR('',#22949,1.);
#6590=VECTOR('',#22950,1.);
#6591=VECTOR('',#22953,1.);
#6592=VECTOR('',#22954,1.);
#6593=VECTOR('',#22955,1.);
#6594=VECTOR('',#22958,1.);
#6595=VECTOR('',#22959,1.);
#6596=VECTOR('',#22964,1.);
#6597=VECTOR('',#22965,1.);
#6598=VECTOR('',#22966,1.);
#6599=VECTOR('',#22967,1.);
#6600=VECTOR('',#22970,1.);
#6601=VECTOR('',#22971,1.);
#6602=VECTOR('',#22972,1.);
#6603=VECTOR('',#22975,1.);
#6604=VECTOR('',#22976,1.);
#6605=VECTOR('',#22977,1.);
#6606=VECTOR('',#22980,1.);
#6607=VECTOR('',#22981,1.);
#6608=VECTOR('',#22986,1.);
#6609=VECTOR('',#22987,1.);
#6610=VECTOR('',#22988,1.);
#6611=VECTOR('',#22989,1.);
#6612=VECTOR('',#22992,1.);
#6613=VECTOR('',#22993,1.);
#6614=VECTOR('',#22994,1.);
#6615=VECTOR('',#22997,1.);
#6616=VECTOR('',#22998,1.);
#6617=VECTOR('',#22999,1.);
#6618=VECTOR('',#23002,1.);
#6619=VECTOR('',#23003,1.);
#6620=VECTOR('',#23008,1.);
#6621=VECTOR('',#23009,1.);
#6622=VECTOR('',#23010,1.);
#6623=VECTOR('',#23011,1.);
#6624=VECTOR('',#23014,1.);
#6625=VECTOR('',#23015,1.);
#6626=VECTOR('',#23016,1.);
#6627=VECTOR('',#23019,1.);
#6628=VECTOR('',#23020,1.);
#6629=VECTOR('',#23021,1.);
#6630=VECTOR('',#23024,1.);
#6631=VECTOR('',#23025,1.);
#6632=VECTOR('',#23030,1.);
#6633=VECTOR('',#23031,1.);
#6634=VECTOR('',#23032,1.);
#6635=VECTOR('',#23033,1.);
#6636=VECTOR('',#23036,1.);
#6637=VECTOR('',#23037,1.);
#6638=VECTOR('',#23038,1.);
#6639=VECTOR('',#23041,1.);
#6640=VECTOR('',#23042,1.);
#6641=VECTOR('',#23043,1.);
#6642=VECTOR('',#23046,1.);
#6643=VECTOR('',#23047,1.);
#6644=VECTOR('',#23054,0.274999999999999);
#6645=VECTOR('',#23061,0.275);
#6646=VECTOR('',#23066,1.);
#6647=VECTOR('',#23067,1.);
#6648=VECTOR('',#23068,1.);
#6649=VECTOR('',#23069,1.);
#6650=VECTOR('',#23072,1.);
#6651=VECTOR('',#23073,1.);
#6652=VECTOR('',#23074,1.);
#6653=VECTOR('',#23077,1.);
#6654=VECTOR('',#23078,1.);
#6655=VECTOR('',#23079,1.);
#6656=VECTOR('',#23082,1.);
#6657=VECTOR('',#23083,1.);
#7698=CIRCLE('',#19909,0.274999999999999);
#7699=CIRCLE('',#19910,0.274999999999999);
#7700=CIRCLE('',#19912,0.275);
#7701=CIRCLE('',#19913,0.275);
#8492=VERTEX_POINT('',#27614);
#8493=VERTEX_POINT('',#27615);
#8494=VERTEX_POINT('',#27617);
#8495=VERTEX_POINT('',#27619);
#8496=VERTEX_POINT('',#27623);
#8497=VERTEX_POINT('',#27625);
#8498=VERTEX_POINT('',#27629);
#8499=VERTEX_POINT('',#27631);
#8500=VERTEX_POINT('',#27639);
#8501=VERTEX_POINT('',#27640);
#8502=VERTEX_POINT('',#27642);
#8503=VERTEX_POINT('',#27644);
#8504=VERTEX_POINT('',#27648);
#8505=VERTEX_POINT('',#27650);
#8506=VERTEX_POINT('',#27654);
#8507=VERTEX_POINT('',#27656);
#8508=VERTEX_POINT('',#27664);
#8509=VERTEX_POINT('',#27665);
#8510=VERTEX_POINT('',#27667);
#8511=VERTEX_POINT('',#27669);
#8512=VERTEX_POINT('',#27673);
#8513=VERTEX_POINT('',#27675);
#8514=VERTEX_POINT('',#27679);
#8515=VERTEX_POINT('',#27681);
#8516=VERTEX_POINT('',#27689);
#8517=VERTEX_POINT('',#27690);
#8518=VERTEX_POINT('',#27692);
#8519=VERTEX_POINT('',#27694);
#8520=VERTEX_POINT('',#27698);
#8521=VERTEX_POINT('',#27700);
#8522=VERTEX_POINT('',#27704);
#8523=VERTEX_POINT('',#27706);
#8524=VERTEX_POINT('',#27714);
#8525=VERTEX_POINT('',#27715);
#8526=VERTEX_POINT('',#27717);
#8527=VERTEX_POINT('',#27719);
#8528=VERTEX_POINT('',#27723);
#8529=VERTEX_POINT('',#27725);
#8530=VERTEX_POINT('',#27729);
#8531=VERTEX_POINT('',#27731);
#8532=VERTEX_POINT('',#27739);
#8533=VERTEX_POINT('',#27740);
#8534=VERTEX_POINT('',#27742);
#8535=VERTEX_POINT('',#27744);
#8536=VERTEX_POINT('',#27748);
#8537=VERTEX_POINT('',#27750);
#8538=VERTEX_POINT('',#27754);
#8539=VERTEX_POINT('',#27756);
#8540=VERTEX_POINT('',#27764);
#8541=VERTEX_POINT('',#27765);
#8542=VERTEX_POINT('',#27767);
#8543=VERTEX_POINT('',#27769);
#8544=VERTEX_POINT('',#27773);
#8545=VERTEX_POINT('',#27775);
#8546=VERTEX_POINT('',#27779);
#8547=VERTEX_POINT('',#27781);
#8548=VERTEX_POINT('',#27789);
#8549=VERTEX_POINT('',#27790);
#8550=VERTEX_POINT('',#27792);
#8551=VERTEX_POINT('',#27794);
#8552=VERTEX_POINT('',#27798);
#8553=VERTEX_POINT('',#27800);
#8554=VERTEX_POINT('',#27804);
#8555=VERTEX_POINT('',#27806);
#8556=VERTEX_POINT('',#27814);
#8557=VERTEX_POINT('',#27815);
#8558=VERTEX_POINT('',#27817);
#8559=VERTEX_POINT('',#27819);
#8560=VERTEX_POINT('',#27823);
#8561=VERTEX_POINT('',#27825);
#8562=VERTEX_POINT('',#27829);
#8563=VERTEX_POINT('',#27831);
#8564=VERTEX_POINT('',#27839);
#8565=VERTEX_POINT('',#27840);
#8566=VERTEX_POINT('',#27842);
#8567=VERTEX_POINT('',#27844);
#8568=VERTEX_POINT('',#27848);
#8569=VERTEX_POINT('',#27850);
#8570=VERTEX_POINT('',#27854);
#8571=VERTEX_POINT('',#27856);
#8572=VERTEX_POINT('',#27864);
#8573=VERTEX_POINT('',#27865);
#8574=VERTEX_POINT('',#27867);
#8575=VERTEX_POINT('',#27869);
#8576=VERTEX_POINT('',#27873);
#8577=VERTEX_POINT('',#27875);
#8578=VERTEX_POINT('',#27879);
#8579=VERTEX_POINT('',#27881);
#8580=VERTEX_POINT('',#27889);
#8581=VERTEX_POINT('',#27890);
#8582=VERTEX_POINT('',#27892);
#8583=VERTEX_POINT('',#27894);
#8584=VERTEX_POINT('',#27898);
#8585=VERTEX_POINT('',#27900);
#8586=VERTEX_POINT('',#27904);
#8587=VERTEX_POINT('',#27906);
#8588=VERTEX_POINT('',#27914);
#8589=VERTEX_POINT('',#27915);
#8590=VERTEX_POINT('',#27917);
#8591=VERTEX_POINT('',#27919);
#8592=VERTEX_POINT('',#27923);
#8593=VERTEX_POINT('',#27925);
#8594=VERTEX_POINT('',#27929);
#8595=VERTEX_POINT('',#27931);
#8596=VERTEX_POINT('',#27939);
#8597=VERTEX_POINT('',#27940);
#8598=VERTEX_POINT('',#27942);
#8599=VERTEX_POINT('',#27944);
#8600=VERTEX_POINT('',#27948);
#8601=VERTEX_POINT('',#27950);
#8602=VERTEX_POINT('',#27954);
#8603=VERTEX_POINT('',#27956);
#8604=VERTEX_POINT('',#27964);
#8605=VERTEX_POINT('',#27965);
#8606=VERTEX_POINT('',#27967);
#8607=VERTEX_POINT('',#27969);
#8608=VERTEX_POINT('',#27973);
#8609=VERTEX_POINT('',#27975);
#8610=VERTEX_POINT('',#27979);
#8611=VERTEX_POINT('',#27981);
#8612=VERTEX_POINT('',#27989);
#8613=VERTEX_POINT('',#27990);
#8614=VERTEX_POINT('',#27992);
#8615=VERTEX_POINT('',#27994);
#8616=VERTEX_POINT('',#27998);
#8617=VERTEX_POINT('',#28000);
#8618=VERTEX_POINT('',#28004);
#8619=VERTEX_POINT('',#28006);
#8620=VERTEX_POINT('',#28014);
#8621=VERTEX_POINT('',#28015);
#8622=VERTEX_POINT('',#28017);
#8623=VERTEX_POINT('',#28019);
#8624=VERTEX_POINT('',#28023);
#8625=VERTEX_POINT('',#28025);
#8626=VERTEX_POINT('',#28029);
#8627=VERTEX_POINT('',#28031);
#8628=VERTEX_POINT('',#28039);
#8629=VERTEX_POINT('',#28040);
#8630=VERTEX_POINT('',#28042);
#8631=VERTEX_POINT('',#28044);
#8632=VERTEX_POINT('',#28048);
#8633=VERTEX_POINT('',#28050);
#8634=VERTEX_POINT('',#28054);
#8635=VERTEX_POINT('',#28056);
#8636=VERTEX_POINT('',#28064);
#8637=VERTEX_POINT('',#28065);
#8638=VERTEX_POINT('',#28067);
#8639=VERTEX_POINT('',#28069);
#8640=VERTEX_POINT('',#28073);
#8641=VERTEX_POINT('',#28075);
#8642=VERTEX_POINT('',#28079);
#8643=VERTEX_POINT('',#28081);
#8644=VERTEX_POINT('',#28089);
#8645=VERTEX_POINT('',#28090);
#8646=VERTEX_POINT('',#28092);
#8647=VERTEX_POINT('',#28094);
#8648=VERTEX_POINT('',#28098);
#8649=VERTEX_POINT('',#28100);
#8650=VERTEX_POINT('',#28104);
#8651=VERTEX_POINT('',#28106);
#8652=VERTEX_POINT('',#28114);
#8653=VERTEX_POINT('',#28115);
#8654=VERTEX_POINT('',#28117);
#8655=VERTEX_POINT('',#28119);
#8656=VERTEX_POINT('',#28123);
#8657=VERTEX_POINT('',#28125);
#8658=VERTEX_POINT('',#28129);
#8659=VERTEX_POINT('',#28131);
#8660=VERTEX_POINT('',#28139);
#8661=VERTEX_POINT('',#28140);
#8662=VERTEX_POINT('',#28142);
#8663=VERTEX_POINT('',#28144);
#8664=VERTEX_POINT('',#28148);
#8665=VERTEX_POINT('',#28150);
#8666=VERTEX_POINT('',#28154);
#8667=VERTEX_POINT('',#28156);
#8668=VERTEX_POINT('',#28164);
#8669=VERTEX_POINT('',#28165);
#8670=VERTEX_POINT('',#28167);
#8671=VERTEX_POINT('',#28169);
#8672=VERTEX_POINT('',#28173);
#8673=VERTEX_POINT('',#28175);
#8674=VERTEX_POINT('',#28179);
#8675=VERTEX_POINT('',#28181);
#8676=VERTEX_POINT('',#28189);
#8677=VERTEX_POINT('',#28190);
#8678=VERTEX_POINT('',#28192);
#8679=VERTEX_POINT('',#28194);
#8680=VERTEX_POINT('',#28198);
#8681=VERTEX_POINT('',#28200);
#8682=VERTEX_POINT('',#28204);
#8683=VERTEX_POINT('',#28206);
#8684=VERTEX_POINT('',#28214);
#8685=VERTEX_POINT('',#28215);
#8686=VERTEX_POINT('',#28217);
#8687=VERTEX_POINT('',#28219);
#8688=VERTEX_POINT('',#28223);
#8689=VERTEX_POINT('',#28225);
#8690=VERTEX_POINT('',#28229);
#8691=VERTEX_POINT('',#28231);
#8692=VERTEX_POINT('',#28239);
#8693=VERTEX_POINT('',#28241);
#8694=VERTEX_POINT('',#28245);
#8695=VERTEX_POINT('',#28247);
#8696=VERTEX_POINT('',#28251);
#8697=VERTEX_POINT('',#28252);
#8698=VERTEX_POINT('',#28254);
#8699=VERTEX_POINT('',#28256);
#8700=VERTEX_POINT('',#28260);
#8701=VERTEX_POINT('',#28262);
#8702=VERTEX_POINT('',#28266);
#8703=VERTEX_POINT('',#28268);
#10307=EDGE_CURVE('',#8492,#8493,#4912,.T.);
#10308=EDGE_CURVE('',#8492,#8494,#4913,.T.);
#10309=EDGE_CURVE('',#8494,#8495,#4914,.T.);
#10310=EDGE_CURVE('',#8493,#8495,#4915,.T.);
#10311=EDGE_CURVE('',#8493,#8496,#4916,.T.);
#10312=EDGE_CURVE('',#8495,#8497,#4917,.T.);
#10313=EDGE_CURVE('',#8496,#8497,#4918,.T.);
#10314=EDGE_CURVE('',#8496,#8498,#4919,.T.);
#10315=EDGE_CURVE('',#8497,#8499,#4920,.T.);
#10316=EDGE_CURVE('',#8498,#8499,#4921,.T.);
#10317=EDGE_CURVE('',#8498,#8492,#4922,.T.);
#10318=EDGE_CURVE('',#8499,#8494,#4923,.T.);
#10319=EDGE_CURVE('',#8500,#8501,#4924,.T.);
#10320=EDGE_CURVE('',#8500,#8502,#4925,.T.);
#10321=EDGE_CURVE('',#8502,#8503,#4926,.T.);
#10322=EDGE_CURVE('',#8501,#8503,#4927,.T.);
#10323=EDGE_CURVE('',#8501,#8504,#4928,.T.);
#10324=EDGE_CURVE('',#8503,#8505,#4929,.T.);
#10325=EDGE_CURVE('',#8504,#8505,#4930,.T.);
#10326=EDGE_CURVE('',#8504,#8506,#4931,.T.);
#10327=EDGE_CURVE('',#8505,#8507,#4932,.T.);
#10328=EDGE_CURVE('',#8506,#8507,#4933,.T.);
#10329=EDGE_CURVE('',#8506,#8500,#4934,.T.);
#10330=EDGE_CURVE('',#8507,#8502,#4935,.T.);
#10331=EDGE_CURVE('',#8508,#8509,#4936,.T.);
#10332=EDGE_CURVE('',#8508,#8510,#4937,.T.);
#10333=EDGE_CURVE('',#8510,#8511,#4938,.T.);
#10334=EDGE_CURVE('',#8509,#8511,#4939,.T.);
#10335=EDGE_CURVE('',#8509,#8512,#4940,.T.);
#10336=EDGE_CURVE('',#8511,#8513,#4941,.T.);
#10337=EDGE_CURVE('',#8512,#8513,#4942,.T.);
#10338=EDGE_CURVE('',#8512,#8514,#4943,.T.);
#10339=EDGE_CURVE('',#8513,#8515,#4944,.T.);
#10340=EDGE_CURVE('',#8514,#8515,#4945,.T.);
#10341=EDGE_CURVE('',#8514,#8508,#4946,.T.);
#10342=EDGE_CURVE('',#8515,#8510,#4947,.T.);
#10343=EDGE_CURVE('',#8516,#8517,#4948,.T.);
#10344=EDGE_CURVE('',#8516,#8518,#4949,.T.);
#10345=EDGE_CURVE('',#8518,#8519,#4950,.T.);
#10346=EDGE_CURVE('',#8517,#8519,#4951,.T.);
#10347=EDGE_CURVE('',#8517,#8520,#4952,.T.);
#10348=EDGE_CURVE('',#8519,#8521,#4953,.T.);
#10349=EDGE_CURVE('',#8520,#8521,#4954,.T.);
#10350=EDGE_CURVE('',#8520,#8522,#4955,.T.);
#10351=EDGE_CURVE('',#8521,#8523,#4956,.T.);
#10352=EDGE_CURVE('',#8522,#8523,#4957,.T.);
#10353=EDGE_CURVE('',#8522,#8516,#4958,.T.);
#10354=EDGE_CURVE('',#8523,#8518,#4959,.T.);
#10355=EDGE_CURVE('',#8524,#8525,#4960,.T.);
#10356=EDGE_CURVE('',#8524,#8526,#4961,.T.);
#10357=EDGE_CURVE('',#8526,#8527,#4962,.T.);
#10358=EDGE_CURVE('',#8525,#8527,#4963,.T.);
#10359=EDGE_CURVE('',#8525,#8528,#4964,.T.);
#10360=EDGE_CURVE('',#8527,#8529,#4965,.T.);
#10361=EDGE_CURVE('',#8528,#8529,#4966,.T.);
#10362=EDGE_CURVE('',#8528,#8530,#4967,.T.);
#10363=EDGE_CURVE('',#8529,#8531,#4968,.T.);
#10364=EDGE_CURVE('',#8530,#8531,#4969,.T.);
#10365=EDGE_CURVE('',#8530,#8524,#4970,.T.);
#10366=EDGE_CURVE('',#8531,#8526,#4971,.T.);
#10367=EDGE_CURVE('',#8532,#8533,#4972,.T.);
#10368=EDGE_CURVE('',#8532,#8534,#4973,.T.);
#10369=EDGE_CURVE('',#8534,#8535,#4974,.T.);
#10370=EDGE_CURVE('',#8533,#8535,#4975,.T.);
#10371=EDGE_CURVE('',#8533,#8536,#4976,.T.);
#10372=EDGE_CURVE('',#8535,#8537,#4977,.T.);
#10373=EDGE_CURVE('',#8536,#8537,#4978,.T.);
#10374=EDGE_CURVE('',#8536,#8538,#4979,.T.);
#10375=EDGE_CURVE('',#8537,#8539,#4980,.T.);
#10376=EDGE_CURVE('',#8538,#8539,#4981,.T.);
#10377=EDGE_CURVE('',#8538,#8532,#4982,.T.);
#10378=EDGE_CURVE('',#8539,#8534,#4983,.T.);
#10379=EDGE_CURVE('',#8540,#8541,#4984,.T.);
#10380=EDGE_CURVE('',#8540,#8542,#4985,.T.);
#10381=EDGE_CURVE('',#8542,#8543,#4986,.T.);
#10382=EDGE_CURVE('',#8541,#8543,#4987,.T.);
#10383=EDGE_CURVE('',#8541,#8544,#4988,.T.);
#10384=EDGE_CURVE('',#8543,#8545,#4989,.T.);
#10385=EDGE_CURVE('',#8544,#8545,#4990,.T.);
#10386=EDGE_CURVE('',#8544,#8546,#4991,.T.);
#10387=EDGE_CURVE('',#8545,#8547,#4992,.T.);
#10388=EDGE_CURVE('',#8546,#8547,#4993,.T.);
#10389=EDGE_CURVE('',#8546,#8540,#4994,.T.);
#10390=EDGE_CURVE('',#8547,#8542,#4995,.T.);
#10391=EDGE_CURVE('',#8548,#8549,#4996,.T.);
#10392=EDGE_CURVE('',#8548,#8550,#4997,.T.);
#10393=EDGE_CURVE('',#8550,#8551,#4998,.T.);
#10394=EDGE_CURVE('',#8549,#8551,#4999,.T.);
#10395=EDGE_CURVE('',#8549,#8552,#5000,.T.);
#10396=EDGE_CURVE('',#8551,#8553,#5001,.T.);
#10397=EDGE_CURVE('',#8552,#8553,#5002,.T.);
#10398=EDGE_CURVE('',#8552,#8554,#5003,.T.);
#10399=EDGE_CURVE('',#8553,#8555,#5004,.T.);
#10400=EDGE_CURVE('',#8554,#8555,#5005,.T.);
#10401=EDGE_CURVE('',#8554,#8548,#5006,.T.);
#10402=EDGE_CURVE('',#8555,#8550,#5007,.T.);
#10403=EDGE_CURVE('',#8556,#8557,#5008,.T.);
#10404=EDGE_CURVE('',#8556,#8558,#5009,.T.);
#10405=EDGE_CURVE('',#8558,#8559,#5010,.T.);
#10406=EDGE_CURVE('',#8557,#8559,#5011,.T.);
#10407=EDGE_CURVE('',#8557,#8560,#5012,.T.);
#10408=EDGE_CURVE('',#8559,#8561,#5013,.T.);
#10409=EDGE_CURVE('',#8560,#8561,#5014,.T.);
#10410=EDGE_CURVE('',#8560,#8562,#5015,.T.);
#10411=EDGE_CURVE('',#8561,#8563,#5016,.T.);
#10412=EDGE_CURVE('',#8562,#8563,#5017,.T.);
#10413=EDGE_CURVE('',#8562,#8556,#5018,.T.);
#10414=EDGE_CURVE('',#8563,#8558,#5019,.T.);
#10415=EDGE_CURVE('',#8564,#8565,#5020,.T.);
#10416=EDGE_CURVE('',#8564,#8566,#5021,.T.);
#10417=EDGE_CURVE('',#8566,#8567,#5022,.T.);
#10418=EDGE_CURVE('',#8565,#8567,#5023,.T.);
#10419=EDGE_CURVE('',#8565,#8568,#5024,.T.);
#10420=EDGE_CURVE('',#8567,#8569,#5025,.T.);
#10421=EDGE_CURVE('',#8568,#8569,#5026,.T.);
#10422=EDGE_CURVE('',#8568,#8570,#5027,.T.);
#10423=EDGE_CURVE('',#8569,#8571,#5028,.T.);
#10424=EDGE_CURVE('',#8570,#8571,#5029,.T.);
#10425=EDGE_CURVE('',#8570,#8564,#5030,.T.);
#10426=EDGE_CURVE('',#8571,#8566,#5031,.T.);
#10427=EDGE_CURVE('',#8572,#8573,#5032,.T.);
#10428=EDGE_CURVE('',#8572,#8574,#5033,.T.);
#10429=EDGE_CURVE('',#8574,#8575,#5034,.T.);
#10430=EDGE_CURVE('',#8573,#8575,#5035,.T.);
#10431=EDGE_CURVE('',#8573,#8576,#5036,.T.);
#10432=EDGE_CURVE('',#8575,#8577,#5037,.T.);
#10433=EDGE_CURVE('',#8576,#8577,#5038,.T.);
#10434=EDGE_CURVE('',#8576,#8578,#5039,.T.);
#10435=EDGE_CURVE('',#8577,#8579,#5040,.T.);
#10436=EDGE_CURVE('',#8578,#8579,#5041,.T.);
#10437=EDGE_CURVE('',#8578,#8572,#5042,.T.);
#10438=EDGE_CURVE('',#8579,#8574,#5043,.T.);
#10439=EDGE_CURVE('',#8580,#8581,#5044,.T.);
#10440=EDGE_CURVE('',#8580,#8582,#5045,.T.);
#10441=EDGE_CURVE('',#8582,#8583,#5046,.T.);
#10442=EDGE_CURVE('',#8581,#8583,#5047,.T.);
#10443=EDGE_CURVE('',#8581,#8584,#5048,.T.);
#10444=EDGE_CURVE('',#8583,#8585,#5049,.T.);
#10445=EDGE_CURVE('',#8584,#8585,#5050,.T.);
#10446=EDGE_CURVE('',#8584,#8586,#5051,.T.);
#10447=EDGE_CURVE('',#8585,#8587,#5052,.T.);
#10448=EDGE_CURVE('',#8586,#8587,#5053,.T.);
#10449=EDGE_CURVE('',#8586,#8580,#5054,.T.);
#10450=EDGE_CURVE('',#8587,#8582,#5055,.T.);
#10451=EDGE_CURVE('',#8588,#8589,#5056,.T.);
#10452=EDGE_CURVE('',#8588,#8590,#5057,.T.);
#10453=EDGE_CURVE('',#8590,#8591,#5058,.T.);
#10454=EDGE_CURVE('',#8589,#8591,#5059,.T.);
#10455=EDGE_CURVE('',#8589,#8592,#5060,.T.);
#10456=EDGE_CURVE('',#8591,#8593,#5061,.T.);
#10457=EDGE_CURVE('',#8592,#8593,#5062,.T.);
#10458=EDGE_CURVE('',#8592,#8594,#5063,.T.);
#10459=EDGE_CURVE('',#8593,#8595,#5064,.T.);
#10460=EDGE_CURVE('',#8594,#8595,#5065,.T.);
#10461=EDGE_CURVE('',#8594,#8588,#5066,.T.);
#10462=EDGE_CURVE('',#8595,#8590,#5067,.T.);
#10463=EDGE_CURVE('',#8596,#8597,#5068,.T.);
#10464=EDGE_CURVE('',#8596,#8598,#5069,.T.);
#10465=EDGE_CURVE('',#8598,#8599,#5070,.T.);
#10466=EDGE_CURVE('',#8597,#8599,#5071,.T.);
#10467=EDGE_CURVE('',#8597,#8600,#5072,.T.);
#10468=EDGE_CURVE('',#8599,#8601,#5073,.T.);
#10469=EDGE_CURVE('',#8600,#8601,#5074,.T.);
#10470=EDGE_CURVE('',#8600,#8602,#5075,.T.);
#10471=EDGE_CURVE('',#8601,#8603,#5076,.T.);
#10472=EDGE_CURVE('',#8602,#8603,#5077,.T.);
#10473=EDGE_CURVE('',#8602,#8596,#5078,.T.);
#10474=EDGE_CURVE('',#8603,#8598,#5079,.T.);
#10475=EDGE_CURVE('',#8604,#8605,#5080,.T.);
#10476=EDGE_CURVE('',#8604,#8606,#5081,.T.);
#10477=EDGE_CURVE('',#8606,#8607,#5082,.T.);
#10478=EDGE_CURVE('',#8605,#8607,#5083,.T.);
#10479=EDGE_CURVE('',#8605,#8608,#5084,.T.);
#10480=EDGE_CURVE('',#8607,#8609,#5085,.T.);
#10481=EDGE_CURVE('',#8608,#8609,#5086,.T.);
#10482=EDGE_CURVE('',#8608,#8610,#5087,.T.);
#10483=EDGE_CURVE('',#8609,#8611,#5088,.T.);
#10484=EDGE_CURVE('',#8610,#8611,#5089,.T.);
#10485=EDGE_CURVE('',#8610,#8604,#5090,.T.);
#10486=EDGE_CURVE('',#8611,#8606,#5091,.T.);
#10487=EDGE_CURVE('',#8612,#8613,#5092,.T.);
#10488=EDGE_CURVE('',#8612,#8614,#5093,.T.);
#10489=EDGE_CURVE('',#8614,#8615,#5094,.T.);
#10490=EDGE_CURVE('',#8613,#8615,#5095,.T.);
#10491=EDGE_CURVE('',#8613,#8616,#5096,.T.);
#10492=EDGE_CURVE('',#8615,#8617,#5097,.T.);
#10493=EDGE_CURVE('',#8616,#8617,#5098,.T.);
#10494=EDGE_CURVE('',#8616,#8618,#5099,.T.);
#10495=EDGE_CURVE('',#8617,#8619,#5100,.T.);
#10496=EDGE_CURVE('',#8618,#8619,#5101,.T.);
#10497=EDGE_CURVE('',#8618,#8612,#5102,.T.);
#10498=EDGE_CURVE('',#8619,#8614,#5103,.T.);
#10499=EDGE_CURVE('',#8620,#8621,#5104,.T.);
#10500=EDGE_CURVE('',#8620,#8622,#5105,.T.);
#10501=EDGE_CURVE('',#8622,#8623,#5106,.T.);
#10502=EDGE_CURVE('',#8621,#8623,#5107,.T.);
#10503=EDGE_CURVE('',#8621,#8624,#5108,.T.);
#10504=EDGE_CURVE('',#8623,#8625,#5109,.T.);
#10505=EDGE_CURVE('',#8624,#8625,#5110,.T.);
#10506=EDGE_CURVE('',#8624,#8626,#5111,.T.);
#10507=EDGE_CURVE('',#8625,#8627,#5112,.T.);
#10508=EDGE_CURVE('',#8626,#8627,#5113,.T.);
#10509=EDGE_CURVE('',#8626,#8620,#5114,.T.);
#10510=EDGE_CURVE('',#8627,#8622,#5115,.T.);
#10511=EDGE_CURVE('',#8628,#8629,#5116,.T.);
#10512=EDGE_CURVE('',#8628,#8630,#5117,.T.);
#10513=EDGE_CURVE('',#8630,#8631,#5118,.T.);
#10514=EDGE_CURVE('',#8629,#8631,#5119,.T.);
#10515=EDGE_CURVE('',#8629,#8632,#5120,.T.);
#10516=EDGE_CURVE('',#8631,#8633,#5121,.T.);
#10517=EDGE_CURVE('',#8632,#8633,#5122,.T.);
#10518=EDGE_CURVE('',#8632,#8634,#5123,.T.);
#10519=EDGE_CURVE('',#8633,#8635,#5124,.T.);
#10520=EDGE_CURVE('',#8634,#8635,#5125,.T.);
#10521=EDGE_CURVE('',#8634,#8628,#5126,.T.);
#10522=EDGE_CURVE('',#8635,#8630,#5127,.T.);
#10523=EDGE_CURVE('',#8636,#8637,#5128,.T.);
#10524=EDGE_CURVE('',#8636,#8638,#5129,.T.);
#10525=EDGE_CURVE('',#8638,#8639,#5130,.T.);
#10526=EDGE_CURVE('',#8637,#8639,#5131,.T.);
#10527=EDGE_CURVE('',#8637,#8640,#5132,.T.);
#10528=EDGE_CURVE('',#8639,#8641,#5133,.T.);
#10529=EDGE_CURVE('',#8640,#8641,#5134,.T.);
#10530=EDGE_CURVE('',#8640,#8642,#5135,.T.);
#10531=EDGE_CURVE('',#8641,#8643,#5136,.T.);
#10532=EDGE_CURVE('',#8642,#8643,#5137,.T.);
#10533=EDGE_CURVE('',#8642,#8636,#5138,.T.);
#10534=EDGE_CURVE('',#8643,#8638,#5139,.T.);
#10535=EDGE_CURVE('',#8644,#8645,#5140,.T.);
#10536=EDGE_CURVE('',#8644,#8646,#5141,.T.);
#10537=EDGE_CURVE('',#8646,#8647,#5142,.T.);
#10538=EDGE_CURVE('',#8645,#8647,#5143,.T.);
#10539=EDGE_CURVE('',#8645,#8648,#5144,.T.);
#10540=EDGE_CURVE('',#8647,#8649,#5145,.T.);
#10541=EDGE_CURVE('',#8648,#8649,#5146,.T.);
#10542=EDGE_CURVE('',#8648,#8650,#5147,.T.);
#10543=EDGE_CURVE('',#8649,#8651,#5148,.T.);
#10544=EDGE_CURVE('',#8650,#8651,#5149,.T.);
#10545=EDGE_CURVE('',#8650,#8644,#5150,.T.);
#10546=EDGE_CURVE('',#8651,#8646,#5151,.T.);
#10547=EDGE_CURVE('',#8652,#8653,#5152,.T.);
#10548=EDGE_CURVE('',#8652,#8654,#5153,.T.);
#10549=EDGE_CURVE('',#8654,#8655,#5154,.T.);
#10550=EDGE_CURVE('',#8653,#8655,#5155,.T.);
#10551=EDGE_CURVE('',#8653,#8656,#5156,.T.);
#10552=EDGE_CURVE('',#8655,#8657,#5157,.T.);
#10553=EDGE_CURVE('',#8656,#8657,#5158,.T.);
#10554=EDGE_CURVE('',#8656,#8658,#5159,.T.);
#10555=EDGE_CURVE('',#8657,#8659,#5160,.T.);
#10556=EDGE_CURVE('',#8658,#8659,#5161,.T.);
#10557=EDGE_CURVE('',#8658,#8652,#5162,.T.);
#10558=EDGE_CURVE('',#8659,#8654,#5163,.T.);
#10559=EDGE_CURVE('',#8660,#8661,#5164,.T.);
#10560=EDGE_CURVE('',#8660,#8662,#5165,.T.);
#10561=EDGE_CURVE('',#8662,#8663,#5166,.T.);
#10562=EDGE_CURVE('',#8661,#8663,#5167,.T.);
#10563=EDGE_CURVE('',#8661,#8664,#5168,.T.);
#10564=EDGE_CURVE('',#8663,#8665,#5169,.T.);
#10565=EDGE_CURVE('',#8664,#8665,#5170,.T.);
#10566=EDGE_CURVE('',#8664,#8666,#5171,.T.);
#10567=EDGE_CURVE('',#8665,#8667,#5172,.T.);
#10568=EDGE_CURVE('',#8666,#8667,#5173,.T.);
#10569=EDGE_CURVE('',#8666,#8660,#5174,.T.);
#10570=EDGE_CURVE('',#8667,#8662,#5175,.T.);
#10571=EDGE_CURVE('',#8668,#8669,#5176,.T.);
#10572=EDGE_CURVE('',#8668,#8670,#5177,.T.);
#10573=EDGE_CURVE('',#8670,#8671,#5178,.T.);
#10574=EDGE_CURVE('',#8669,#8671,#5179,.T.);
#10575=EDGE_CURVE('',#8669,#8672,#5180,.T.);
#10576=EDGE_CURVE('',#8671,#8673,#5181,.T.);
#10577=EDGE_CURVE('',#8672,#8673,#5182,.T.);
#10578=EDGE_CURVE('',#8672,#8674,#5183,.T.);
#10579=EDGE_CURVE('',#8673,#8675,#5184,.T.);
#10580=EDGE_CURVE('',#8674,#8675,#5185,.T.);
#10581=EDGE_CURVE('',#8674,#8668,#5186,.T.);
#10582=EDGE_CURVE('',#8675,#8670,#5187,.T.);
#10583=EDGE_CURVE('',#8676,#8677,#5188,.T.);
#10584=EDGE_CURVE('',#8676,#8678,#5189,.T.);
#10585=EDGE_CURVE('',#8678,#8679,#5190,.T.);
#10586=EDGE_CURVE('',#8677,#8679,#5191,.T.);
#10587=EDGE_CURVE('',#8677,#8680,#5192,.T.);
#10588=EDGE_CURVE('',#8679,#8681,#5193,.T.);
#10589=EDGE_CURVE('',#8680,#8681,#5194,.T.);
#10590=EDGE_CURVE('',#8680,#8682,#5195,.T.);
#10591=EDGE_CURVE('',#8681,#8683,#5196,.T.);
#10592=EDGE_CURVE('',#8682,#8683,#5197,.T.);
#10593=EDGE_CURVE('',#8682,#8676,#5198,.T.);
#10594=EDGE_CURVE('',#8683,#8678,#5199,.T.);
#10595=EDGE_CURVE('',#8684,#8685,#5200,.T.);
#10596=EDGE_CURVE('',#8684,#8686,#5201,.T.);
#10597=EDGE_CURVE('',#8686,#8687,#5202,.T.);
#10598=EDGE_CURVE('',#8685,#8687,#5203,.T.);
#10599=EDGE_CURVE('',#8685,#8688,#5204,.T.);
#10600=EDGE_CURVE('',#8687,#8689,#5205,.T.);
#10601=EDGE_CURVE('',#8688,#8689,#5206,.T.);
#10602=EDGE_CURVE('',#8688,#8690,#5207,.T.);
#10603=EDGE_CURVE('',#8689,#8691,#5208,.T.);
#10604=EDGE_CURVE('',#8690,#8691,#5209,.T.);
#10605=EDGE_CURVE('',#8690,#8684,#5210,.T.);
#10606=EDGE_CURVE('',#8691,#8686,#5211,.T.);
#10607=EDGE_CURVE('',#8692,#8692,#7698,.T.);
#10608=EDGE_CURVE('',#8692,#8693,#5212,.T.);
#10609=EDGE_CURVE('',#8693,#8693,#7699,.T.);
#10610=EDGE_CURVE('',#8694,#8694,#7700,.T.);
#10611=EDGE_CURVE('',#8694,#8695,#5213,.T.);
#10612=EDGE_CURVE('',#8695,#8695,#7701,.T.);
#10613=EDGE_CURVE('',#8696,#8697,#5214,.T.);
#10614=EDGE_CURVE('',#8697,#8698,#5215,.T.);
#10615=EDGE_CURVE('',#8699,#8698,#5216,.T.);
#10616=EDGE_CURVE('',#8696,#8699,#5217,.T.);
#10617=EDGE_CURVE('',#8700,#8696,#5218,.T.);
#10618=EDGE_CURVE('',#8701,#8699,#5219,.T.);
#10619=EDGE_CURVE('',#8700,#8701,#5220,.T.);
#10620=EDGE_CURVE('',#8702,#8700,#5221,.T.);
#10621=EDGE_CURVE('',#8703,#8701,#5222,.T.);
#10622=EDGE_CURVE('',#8702,#8703,#5223,.T.);
#10623=EDGE_CURVE('',#8697,#8702,#5224,.T.);
#10624=EDGE_CURVE('',#8698,#8703,#5225,.T.);
#13285=ORIENTED_EDGE('',*,*,#10307,.F.);
#13286=ORIENTED_EDGE('',*,*,#10308,.T.);
#13287=ORIENTED_EDGE('',*,*,#10309,.T.);
#13288=ORIENTED_EDGE('',*,*,#10310,.F.);
#13289=ORIENTED_EDGE('',*,*,#10311,.F.);
#13290=ORIENTED_EDGE('',*,*,#10310,.T.);
#13291=ORIENTED_EDGE('',*,*,#10312,.T.);
#13292=ORIENTED_EDGE('',*,*,#10313,.F.);
#13293=ORIENTED_EDGE('',*,*,#10314,.F.);
#13294=ORIENTED_EDGE('',*,*,#10313,.T.);
#13295=ORIENTED_EDGE('',*,*,#10315,.T.);
#13296=ORIENTED_EDGE('',*,*,#10316,.F.);
#13297=ORIENTED_EDGE('',*,*,#10317,.F.);
#13298=ORIENTED_EDGE('',*,*,#10316,.T.);
#13299=ORIENTED_EDGE('',*,*,#10318,.T.);
#13300=ORIENTED_EDGE('',*,*,#10308,.F.);
#13301=ORIENTED_EDGE('',*,*,#10318,.F.);
#13302=ORIENTED_EDGE('',*,*,#10315,.F.);
#13303=ORIENTED_EDGE('',*,*,#10312,.F.);
#13304=ORIENTED_EDGE('',*,*,#10309,.F.);
#13305=ORIENTED_EDGE('',*,*,#10319,.F.);
#13306=ORIENTED_EDGE('',*,*,#10320,.T.);
#13307=ORIENTED_EDGE('',*,*,#10321,.T.);
#13308=ORIENTED_EDGE('',*,*,#10322,.F.);
#13309=ORIENTED_EDGE('',*,*,#10323,.F.);
#13310=ORIENTED_EDGE('',*,*,#10322,.T.);
#13311=ORIENTED_EDGE('',*,*,#10324,.T.);
#13312=ORIENTED_EDGE('',*,*,#10325,.F.);
#13313=ORIENTED_EDGE('',*,*,#10326,.F.);
#13314=ORIENTED_EDGE('',*,*,#10325,.T.);
#13315=ORIENTED_EDGE('',*,*,#10327,.T.);
#13316=ORIENTED_EDGE('',*,*,#10328,.F.);
#13317=ORIENTED_EDGE('',*,*,#10329,.F.);
#13318=ORIENTED_EDGE('',*,*,#10328,.T.);
#13319=ORIENTED_EDGE('',*,*,#10330,.T.);
#13320=ORIENTED_EDGE('',*,*,#10320,.F.);
#13321=ORIENTED_EDGE('',*,*,#10330,.F.);
#13322=ORIENTED_EDGE('',*,*,#10327,.F.);
#13323=ORIENTED_EDGE('',*,*,#10324,.F.);
#13324=ORIENTED_EDGE('',*,*,#10321,.F.);
#13325=ORIENTED_EDGE('',*,*,#10331,.F.);
#13326=ORIENTED_EDGE('',*,*,#10332,.T.);
#13327=ORIENTED_EDGE('',*,*,#10333,.T.);
#13328=ORIENTED_EDGE('',*,*,#10334,.F.);
#13329=ORIENTED_EDGE('',*,*,#10335,.F.);
#13330=ORIENTED_EDGE('',*,*,#10334,.T.);
#13331=ORIENTED_EDGE('',*,*,#10336,.T.);
#13332=ORIENTED_EDGE('',*,*,#10337,.F.);
#13333=ORIENTED_EDGE('',*,*,#10338,.F.);
#13334=ORIENTED_EDGE('',*,*,#10337,.T.);
#13335=ORIENTED_EDGE('',*,*,#10339,.T.);
#13336=ORIENTED_EDGE('',*,*,#10340,.F.);
#13337=ORIENTED_EDGE('',*,*,#10341,.F.);
#13338=ORIENTED_EDGE('',*,*,#10340,.T.);
#13339=ORIENTED_EDGE('',*,*,#10342,.T.);
#13340=ORIENTED_EDGE('',*,*,#10332,.F.);
#13341=ORIENTED_EDGE('',*,*,#10342,.F.);
#13342=ORIENTED_EDGE('',*,*,#10339,.F.);
#13343=ORIENTED_EDGE('',*,*,#10336,.F.);
#13344=ORIENTED_EDGE('',*,*,#10333,.F.);
#13345=ORIENTED_EDGE('',*,*,#10343,.F.);
#13346=ORIENTED_EDGE('',*,*,#10344,.T.);
#13347=ORIENTED_EDGE('',*,*,#10345,.T.);
#13348=ORIENTED_EDGE('',*,*,#10346,.F.);
#13349=ORIENTED_EDGE('',*,*,#10347,.F.);
#13350=ORIENTED_EDGE('',*,*,#10346,.T.);
#13351=ORIENTED_EDGE('',*,*,#10348,.T.);
#13352=ORIENTED_EDGE('',*,*,#10349,.F.);
#13353=ORIENTED_EDGE('',*,*,#10350,.F.);
#13354=ORIENTED_EDGE('',*,*,#10349,.T.);
#13355=ORIENTED_EDGE('',*,*,#10351,.T.);
#13356=ORIENTED_EDGE('',*,*,#10352,.F.);
#13357=ORIENTED_EDGE('',*,*,#10353,.F.);
#13358=ORIENTED_EDGE('',*,*,#10352,.T.);
#13359=ORIENTED_EDGE('',*,*,#10354,.T.);
#13360=ORIENTED_EDGE('',*,*,#10344,.F.);
#13361=ORIENTED_EDGE('',*,*,#10354,.F.);
#13362=ORIENTED_EDGE('',*,*,#10351,.F.);
#13363=ORIENTED_EDGE('',*,*,#10348,.F.);
#13364=ORIENTED_EDGE('',*,*,#10345,.F.);
#13365=ORIENTED_EDGE('',*,*,#10355,.F.);
#13366=ORIENTED_EDGE('',*,*,#10356,.T.);
#13367=ORIENTED_EDGE('',*,*,#10357,.T.);
#13368=ORIENTED_EDGE('',*,*,#10358,.F.);
#13369=ORIENTED_EDGE('',*,*,#10359,.F.);
#13370=ORIENTED_EDGE('',*,*,#10358,.T.);
#13371=ORIENTED_EDGE('',*,*,#10360,.T.);
#13372=ORIENTED_EDGE('',*,*,#10361,.F.);
#13373=ORIENTED_EDGE('',*,*,#10362,.F.);
#13374=ORIENTED_EDGE('',*,*,#10361,.T.);
#13375=ORIENTED_EDGE('',*,*,#10363,.T.);
#13376=ORIENTED_EDGE('',*,*,#10364,.F.);
#13377=ORIENTED_EDGE('',*,*,#10365,.F.);
#13378=ORIENTED_EDGE('',*,*,#10364,.T.);
#13379=ORIENTED_EDGE('',*,*,#10366,.T.);
#13380=ORIENTED_EDGE('',*,*,#10356,.F.);
#13381=ORIENTED_EDGE('',*,*,#10366,.F.);
#13382=ORIENTED_EDGE('',*,*,#10363,.F.);
#13383=ORIENTED_EDGE('',*,*,#10360,.F.);
#13384=ORIENTED_EDGE('',*,*,#10357,.F.);
#13385=ORIENTED_EDGE('',*,*,#10367,.F.);
#13386=ORIENTED_EDGE('',*,*,#10368,.T.);
#13387=ORIENTED_EDGE('',*,*,#10369,.T.);
#13388=ORIENTED_EDGE('',*,*,#10370,.F.);
#13389=ORIENTED_EDGE('',*,*,#10371,.F.);
#13390=ORIENTED_EDGE('',*,*,#10370,.T.);
#13391=ORIENTED_EDGE('',*,*,#10372,.T.);
#13392=ORIENTED_EDGE('',*,*,#10373,.F.);
#13393=ORIENTED_EDGE('',*,*,#10374,.F.);
#13394=ORIENTED_EDGE('',*,*,#10373,.T.);
#13395=ORIENTED_EDGE('',*,*,#10375,.T.);
#13396=ORIENTED_EDGE('',*,*,#10376,.F.);
#13397=ORIENTED_EDGE('',*,*,#10377,.F.);
#13398=ORIENTED_EDGE('',*,*,#10376,.T.);
#13399=ORIENTED_EDGE('',*,*,#10378,.T.);
#13400=ORIENTED_EDGE('',*,*,#10368,.F.);
#13401=ORIENTED_EDGE('',*,*,#10378,.F.);
#13402=ORIENTED_EDGE('',*,*,#10375,.F.);
#13403=ORIENTED_EDGE('',*,*,#10372,.F.);
#13404=ORIENTED_EDGE('',*,*,#10369,.F.);
#13405=ORIENTED_EDGE('',*,*,#10379,.F.);
#13406=ORIENTED_EDGE('',*,*,#10380,.T.);
#13407=ORIENTED_EDGE('',*,*,#10381,.T.);
#13408=ORIENTED_EDGE('',*,*,#10382,.F.);
#13409=ORIENTED_EDGE('',*,*,#10383,.F.);
#13410=ORIENTED_EDGE('',*,*,#10382,.T.);
#13411=ORIENTED_EDGE('',*,*,#10384,.T.);
#13412=ORIENTED_EDGE('',*,*,#10385,.F.);
#13413=ORIENTED_EDGE('',*,*,#10386,.F.);
#13414=ORIENTED_EDGE('',*,*,#10385,.T.);
#13415=ORIENTED_EDGE('',*,*,#10387,.T.);
#13416=ORIENTED_EDGE('',*,*,#10388,.F.);
#13417=ORIENTED_EDGE('',*,*,#10389,.F.);
#13418=ORIENTED_EDGE('',*,*,#10388,.T.);
#13419=ORIENTED_EDGE('',*,*,#10390,.T.);
#13420=ORIENTED_EDGE('',*,*,#10380,.F.);
#13421=ORIENTED_EDGE('',*,*,#10390,.F.);
#13422=ORIENTED_EDGE('',*,*,#10387,.F.);
#13423=ORIENTED_EDGE('',*,*,#10384,.F.);
#13424=ORIENTED_EDGE('',*,*,#10381,.F.);
#13425=ORIENTED_EDGE('',*,*,#10391,.F.);
#13426=ORIENTED_EDGE('',*,*,#10392,.T.);
#13427=ORIENTED_EDGE('',*,*,#10393,.T.);
#13428=ORIENTED_EDGE('',*,*,#10394,.F.);
#13429=ORIENTED_EDGE('',*,*,#10395,.F.);
#13430=ORIENTED_EDGE('',*,*,#10394,.T.);
#13431=ORIENTED_EDGE('',*,*,#10396,.T.);
#13432=ORIENTED_EDGE('',*,*,#10397,.F.);
#13433=ORIENTED_EDGE('',*,*,#10398,.F.);
#13434=ORIENTED_EDGE('',*,*,#10397,.T.);
#13435=ORIENTED_EDGE('',*,*,#10399,.T.);
#13436=ORIENTED_EDGE('',*,*,#10400,.F.);
#13437=ORIENTED_EDGE('',*,*,#10401,.F.);
#13438=ORIENTED_EDGE('',*,*,#10400,.T.);
#13439=ORIENTED_EDGE('',*,*,#10402,.T.);
#13440=ORIENTED_EDGE('',*,*,#10392,.F.);
#13441=ORIENTED_EDGE('',*,*,#10402,.F.);
#13442=ORIENTED_EDGE('',*,*,#10399,.F.);
#13443=ORIENTED_EDGE('',*,*,#10396,.F.);
#13444=ORIENTED_EDGE('',*,*,#10393,.F.);
#13445=ORIENTED_EDGE('',*,*,#10403,.F.);
#13446=ORIENTED_EDGE('',*,*,#10404,.T.);
#13447=ORIENTED_EDGE('',*,*,#10405,.T.);
#13448=ORIENTED_EDGE('',*,*,#10406,.F.);
#13449=ORIENTED_EDGE('',*,*,#10407,.F.);
#13450=ORIENTED_EDGE('',*,*,#10406,.T.);
#13451=ORIENTED_EDGE('',*,*,#10408,.T.);
#13452=ORIENTED_EDGE('',*,*,#10409,.F.);
#13453=ORIENTED_EDGE('',*,*,#10410,.F.);
#13454=ORIENTED_EDGE('',*,*,#10409,.T.);
#13455=ORIENTED_EDGE('',*,*,#10411,.T.);
#13456=ORIENTED_EDGE('',*,*,#10412,.F.);
#13457=ORIENTED_EDGE('',*,*,#10413,.F.);
#13458=ORIENTED_EDGE('',*,*,#10412,.T.);
#13459=ORIENTED_EDGE('',*,*,#10414,.T.);
#13460=ORIENTED_EDGE('',*,*,#10404,.F.);
#13461=ORIENTED_EDGE('',*,*,#10414,.F.);
#13462=ORIENTED_EDGE('',*,*,#10411,.F.);
#13463=ORIENTED_EDGE('',*,*,#10408,.F.);
#13464=ORIENTED_EDGE('',*,*,#10405,.F.);
#13465=ORIENTED_EDGE('',*,*,#10415,.F.);
#13466=ORIENTED_EDGE('',*,*,#10416,.T.);
#13467=ORIENTED_EDGE('',*,*,#10417,.T.);
#13468=ORIENTED_EDGE('',*,*,#10418,.F.);
#13469=ORIENTED_EDGE('',*,*,#10419,.F.);
#13470=ORIENTED_EDGE('',*,*,#10418,.T.);
#13471=ORIENTED_EDGE('',*,*,#10420,.T.);
#13472=ORIENTED_EDGE('',*,*,#10421,.F.);
#13473=ORIENTED_EDGE('',*,*,#10422,.F.);
#13474=ORIENTED_EDGE('',*,*,#10421,.T.);
#13475=ORIENTED_EDGE('',*,*,#10423,.T.);
#13476=ORIENTED_EDGE('',*,*,#10424,.F.);
#13477=ORIENTED_EDGE('',*,*,#10425,.F.);
#13478=ORIENTED_EDGE('',*,*,#10424,.T.);
#13479=ORIENTED_EDGE('',*,*,#10426,.T.);
#13480=ORIENTED_EDGE('',*,*,#10416,.F.);
#13481=ORIENTED_EDGE('',*,*,#10426,.F.);
#13482=ORIENTED_EDGE('',*,*,#10423,.F.);
#13483=ORIENTED_EDGE('',*,*,#10420,.F.);
#13484=ORIENTED_EDGE('',*,*,#10417,.F.);
#13485=ORIENTED_EDGE('',*,*,#10427,.F.);
#13486=ORIENTED_EDGE('',*,*,#10428,.T.);
#13487=ORIENTED_EDGE('',*,*,#10429,.T.);
#13488=ORIENTED_EDGE('',*,*,#10430,.F.);
#13489=ORIENTED_EDGE('',*,*,#10431,.F.);
#13490=ORIENTED_EDGE('',*,*,#10430,.T.);
#13491=ORIENTED_EDGE('',*,*,#10432,.T.);
#13492=ORIENTED_EDGE('',*,*,#10433,.F.);
#13493=ORIENTED_EDGE('',*,*,#10434,.F.);
#13494=ORIENTED_EDGE('',*,*,#10433,.T.);
#13495=ORIENTED_EDGE('',*,*,#10435,.T.);
#13496=ORIENTED_EDGE('',*,*,#10436,.F.);
#13497=ORIENTED_EDGE('',*,*,#10437,.F.);
#13498=ORIENTED_EDGE('',*,*,#10436,.T.);
#13499=ORIENTED_EDGE('',*,*,#10438,.T.);
#13500=ORIENTED_EDGE('',*,*,#10428,.F.);
#13501=ORIENTED_EDGE('',*,*,#10438,.F.);
#13502=ORIENTED_EDGE('',*,*,#10435,.F.);
#13503=ORIENTED_EDGE('',*,*,#10432,.F.);
#13504=ORIENTED_EDGE('',*,*,#10429,.F.);
#13505=ORIENTED_EDGE('',*,*,#10439,.F.);
#13506=ORIENTED_EDGE('',*,*,#10440,.T.);
#13507=ORIENTED_EDGE('',*,*,#10441,.T.);
#13508=ORIENTED_EDGE('',*,*,#10442,.F.);
#13509=ORIENTED_EDGE('',*,*,#10443,.F.);
#13510=ORIENTED_EDGE('',*,*,#10442,.T.);
#13511=ORIENTED_EDGE('',*,*,#10444,.T.);
#13512=ORIENTED_EDGE('',*,*,#10445,.F.);
#13513=ORIENTED_EDGE('',*,*,#10446,.F.);
#13514=ORIENTED_EDGE('',*,*,#10445,.T.);
#13515=ORIENTED_EDGE('',*,*,#10447,.T.);
#13516=ORIENTED_EDGE('',*,*,#10448,.F.);
#13517=ORIENTED_EDGE('',*,*,#10449,.F.);
#13518=ORIENTED_EDGE('',*,*,#10448,.T.);
#13519=ORIENTED_EDGE('',*,*,#10450,.T.);
#13520=ORIENTED_EDGE('',*,*,#10440,.F.);
#13521=ORIENTED_EDGE('',*,*,#10450,.F.);
#13522=ORIENTED_EDGE('',*,*,#10447,.F.);
#13523=ORIENTED_EDGE('',*,*,#10444,.F.);
#13524=ORIENTED_EDGE('',*,*,#10441,.F.);
#13525=ORIENTED_EDGE('',*,*,#10451,.F.);
#13526=ORIENTED_EDGE('',*,*,#10452,.T.);
#13527=ORIENTED_EDGE('',*,*,#10453,.T.);
#13528=ORIENTED_EDGE('',*,*,#10454,.F.);
#13529=ORIENTED_EDGE('',*,*,#10455,.F.);
#13530=ORIENTED_EDGE('',*,*,#10454,.T.);
#13531=ORIENTED_EDGE('',*,*,#10456,.T.);
#13532=ORIENTED_EDGE('',*,*,#10457,.F.);
#13533=ORIENTED_EDGE('',*,*,#10458,.F.);
#13534=ORIENTED_EDGE('',*,*,#10457,.T.);
#13535=ORIENTED_EDGE('',*,*,#10459,.T.);
#13536=ORIENTED_EDGE('',*,*,#10460,.F.);
#13537=ORIENTED_EDGE('',*,*,#10461,.F.);
#13538=ORIENTED_EDGE('',*,*,#10460,.T.);
#13539=ORIENTED_EDGE('',*,*,#10462,.T.);
#13540=ORIENTED_EDGE('',*,*,#10452,.F.);
#13541=ORIENTED_EDGE('',*,*,#10462,.F.);
#13542=ORIENTED_EDGE('',*,*,#10459,.F.);
#13543=ORIENTED_EDGE('',*,*,#10456,.F.);
#13544=ORIENTED_EDGE('',*,*,#10453,.F.);
#13545=ORIENTED_EDGE('',*,*,#10463,.F.);
#13546=ORIENTED_EDGE('',*,*,#10464,.T.);
#13547=ORIENTED_EDGE('',*,*,#10465,.T.);
#13548=ORIENTED_EDGE('',*,*,#10466,.F.);
#13549=ORIENTED_EDGE('',*,*,#10467,.F.);
#13550=ORIENTED_EDGE('',*,*,#10466,.T.);
#13551=ORIENTED_EDGE('',*,*,#10468,.T.);
#13552=ORIENTED_EDGE('',*,*,#10469,.F.);
#13553=ORIENTED_EDGE('',*,*,#10470,.F.);
#13554=ORIENTED_EDGE('',*,*,#10469,.T.);
#13555=ORIENTED_EDGE('',*,*,#10471,.T.);
#13556=ORIENTED_EDGE('',*,*,#10472,.F.);
#13557=ORIENTED_EDGE('',*,*,#10473,.F.);
#13558=ORIENTED_EDGE('',*,*,#10472,.T.);
#13559=ORIENTED_EDGE('',*,*,#10474,.T.);
#13560=ORIENTED_EDGE('',*,*,#10464,.F.);
#13561=ORIENTED_EDGE('',*,*,#10474,.F.);
#13562=ORIENTED_EDGE('',*,*,#10471,.F.);
#13563=ORIENTED_EDGE('',*,*,#10468,.F.);
#13564=ORIENTED_EDGE('',*,*,#10465,.F.);
#13565=ORIENTED_EDGE('',*,*,#10475,.F.);
#13566=ORIENTED_EDGE('',*,*,#10476,.T.);
#13567=ORIENTED_EDGE('',*,*,#10477,.T.);
#13568=ORIENTED_EDGE('',*,*,#10478,.F.);
#13569=ORIENTED_EDGE('',*,*,#10479,.F.);
#13570=ORIENTED_EDGE('',*,*,#10478,.T.);
#13571=ORIENTED_EDGE('',*,*,#10480,.T.);
#13572=ORIENTED_EDGE('',*,*,#10481,.F.);
#13573=ORIENTED_EDGE('',*,*,#10482,.F.);
#13574=ORIENTED_EDGE('',*,*,#10481,.T.);
#13575=ORIENTED_EDGE('',*,*,#10483,.T.);
#13576=ORIENTED_EDGE('',*,*,#10484,.F.);
#13577=ORIENTED_EDGE('',*,*,#10485,.F.);
#13578=ORIENTED_EDGE('',*,*,#10484,.T.);
#13579=ORIENTED_EDGE('',*,*,#10486,.T.);
#13580=ORIENTED_EDGE('',*,*,#10476,.F.);
#13581=ORIENTED_EDGE('',*,*,#10486,.F.);
#13582=ORIENTED_EDGE('',*,*,#10483,.F.);
#13583=ORIENTED_EDGE('',*,*,#10480,.F.);
#13584=ORIENTED_EDGE('',*,*,#10477,.F.);
#13585=ORIENTED_EDGE('',*,*,#10487,.F.);
#13586=ORIENTED_EDGE('',*,*,#10488,.T.);
#13587=ORIENTED_EDGE('',*,*,#10489,.T.);
#13588=ORIENTED_EDGE('',*,*,#10490,.F.);
#13589=ORIENTED_EDGE('',*,*,#10491,.F.);
#13590=ORIENTED_EDGE('',*,*,#10490,.T.);
#13591=ORIENTED_EDGE('',*,*,#10492,.T.);
#13592=ORIENTED_EDGE('',*,*,#10493,.F.);
#13593=ORIENTED_EDGE('',*,*,#10494,.F.);
#13594=ORIENTED_EDGE('',*,*,#10493,.T.);
#13595=ORIENTED_EDGE('',*,*,#10495,.T.);
#13596=ORIENTED_EDGE('',*,*,#10496,.F.);
#13597=ORIENTED_EDGE('',*,*,#10497,.F.);
#13598=ORIENTED_EDGE('',*,*,#10496,.T.);
#13599=ORIENTED_EDGE('',*,*,#10498,.T.);
#13600=ORIENTED_EDGE('',*,*,#10488,.F.);
#13601=ORIENTED_EDGE('',*,*,#10498,.F.);
#13602=ORIENTED_EDGE('',*,*,#10495,.F.);
#13603=ORIENTED_EDGE('',*,*,#10492,.F.);
#13604=ORIENTED_EDGE('',*,*,#10489,.F.);
#13605=ORIENTED_EDGE('',*,*,#10499,.F.);
#13606=ORIENTED_EDGE('',*,*,#10500,.T.);
#13607=ORIENTED_EDGE('',*,*,#10501,.T.);
#13608=ORIENTED_EDGE('',*,*,#10502,.F.);
#13609=ORIENTED_EDGE('',*,*,#10503,.F.);
#13610=ORIENTED_EDGE('',*,*,#10502,.T.);
#13611=ORIENTED_EDGE('',*,*,#10504,.T.);
#13612=ORIENTED_EDGE('',*,*,#10505,.F.);
#13613=ORIENTED_EDGE('',*,*,#10506,.F.);
#13614=ORIENTED_EDGE('',*,*,#10505,.T.);
#13615=ORIENTED_EDGE('',*,*,#10507,.T.);
#13616=ORIENTED_EDGE('',*,*,#10508,.F.);
#13617=ORIENTED_EDGE('',*,*,#10509,.F.);
#13618=ORIENTED_EDGE('',*,*,#10508,.T.);
#13619=ORIENTED_EDGE('',*,*,#10510,.T.);
#13620=ORIENTED_EDGE('',*,*,#10500,.F.);
#13621=ORIENTED_EDGE('',*,*,#10510,.F.);
#13622=ORIENTED_EDGE('',*,*,#10507,.F.);
#13623=ORIENTED_EDGE('',*,*,#10504,.F.);
#13624=ORIENTED_EDGE('',*,*,#10501,.F.);
#13625=ORIENTED_EDGE('',*,*,#10511,.F.);
#13626=ORIENTED_EDGE('',*,*,#10512,.T.);
#13627=ORIENTED_EDGE('',*,*,#10513,.T.);
#13628=ORIENTED_EDGE('',*,*,#10514,.F.);
#13629=ORIENTED_EDGE('',*,*,#10515,.F.);
#13630=ORIENTED_EDGE('',*,*,#10514,.T.);
#13631=ORIENTED_EDGE('',*,*,#10516,.T.);
#13632=ORIENTED_EDGE('',*,*,#10517,.F.);
#13633=ORIENTED_EDGE('',*,*,#10518,.F.);
#13634=ORIENTED_EDGE('',*,*,#10517,.T.);
#13635=ORIENTED_EDGE('',*,*,#10519,.T.);
#13636=ORIENTED_EDGE('',*,*,#10520,.F.);
#13637=ORIENTED_EDGE('',*,*,#10521,.F.);
#13638=ORIENTED_EDGE('',*,*,#10520,.T.);
#13639=ORIENTED_EDGE('',*,*,#10522,.T.);
#13640=ORIENTED_EDGE('',*,*,#10512,.F.);
#13641=ORIENTED_EDGE('',*,*,#10522,.F.);
#13642=ORIENTED_EDGE('',*,*,#10519,.F.);
#13643=ORIENTED_EDGE('',*,*,#10516,.F.);
#13644=ORIENTED_EDGE('',*,*,#10513,.F.);
#13645=ORIENTED_EDGE('',*,*,#10523,.F.);
#13646=ORIENTED_EDGE('',*,*,#10524,.T.);
#13647=ORIENTED_EDGE('',*,*,#10525,.T.);
#13648=ORIENTED_EDGE('',*,*,#10526,.F.);
#13649=ORIENTED_EDGE('',*,*,#10527,.F.);
#13650=ORIENTED_EDGE('',*,*,#10526,.T.);
#13651=ORIENTED_EDGE('',*,*,#10528,.T.);
#13652=ORIENTED_EDGE('',*,*,#10529,.F.);
#13653=ORIENTED_EDGE('',*,*,#10530,.F.);
#13654=ORIENTED_EDGE('',*,*,#10529,.T.);
#13655=ORIENTED_EDGE('',*,*,#10531,.T.);
#13656=ORIENTED_EDGE('',*,*,#10532,.F.);
#13657=ORIENTED_EDGE('',*,*,#10533,.F.);
#13658=ORIENTED_EDGE('',*,*,#10532,.T.);
#13659=ORIENTED_EDGE('',*,*,#10534,.T.);
#13660=ORIENTED_EDGE('',*,*,#10524,.F.);
#13661=ORIENTED_EDGE('',*,*,#10534,.F.);
#13662=ORIENTED_EDGE('',*,*,#10531,.F.);
#13663=ORIENTED_EDGE('',*,*,#10528,.F.);
#13664=ORIENTED_EDGE('',*,*,#10525,.F.);
#13665=ORIENTED_EDGE('',*,*,#10535,.F.);
#13666=ORIENTED_EDGE('',*,*,#10536,.T.);
#13667=ORIENTED_EDGE('',*,*,#10537,.T.);
#13668=ORIENTED_EDGE('',*,*,#10538,.F.);
#13669=ORIENTED_EDGE('',*,*,#10539,.F.);
#13670=ORIENTED_EDGE('',*,*,#10538,.T.);
#13671=ORIENTED_EDGE('',*,*,#10540,.T.);
#13672=ORIENTED_EDGE('',*,*,#10541,.F.);
#13673=ORIENTED_EDGE('',*,*,#10542,.F.);
#13674=ORIENTED_EDGE('',*,*,#10541,.T.);
#13675=ORIENTED_EDGE('',*,*,#10543,.T.);
#13676=ORIENTED_EDGE('',*,*,#10544,.F.);
#13677=ORIENTED_EDGE('',*,*,#10545,.F.);
#13678=ORIENTED_EDGE('',*,*,#10544,.T.);
#13679=ORIENTED_EDGE('',*,*,#10546,.T.);
#13680=ORIENTED_EDGE('',*,*,#10536,.F.);
#13681=ORIENTED_EDGE('',*,*,#10546,.F.);
#13682=ORIENTED_EDGE('',*,*,#10543,.F.);
#13683=ORIENTED_EDGE('',*,*,#10540,.F.);
#13684=ORIENTED_EDGE('',*,*,#10537,.F.);
#13685=ORIENTED_EDGE('',*,*,#10547,.F.);
#13686=ORIENTED_EDGE('',*,*,#10548,.T.);
#13687=ORIENTED_EDGE('',*,*,#10549,.T.);
#13688=ORIENTED_EDGE('',*,*,#10550,.F.);
#13689=ORIENTED_EDGE('',*,*,#10551,.F.);
#13690=ORIENTED_EDGE('',*,*,#10550,.T.);
#13691=ORIENTED_EDGE('',*,*,#10552,.T.);
#13692=ORIENTED_EDGE('',*,*,#10553,.F.);
#13693=ORIENTED_EDGE('',*,*,#10554,.F.);
#13694=ORIENTED_EDGE('',*,*,#10553,.T.);
#13695=ORIENTED_EDGE('',*,*,#10555,.T.);
#13696=ORIENTED_EDGE('',*,*,#10556,.F.);
#13697=ORIENTED_EDGE('',*,*,#10557,.F.);
#13698=ORIENTED_EDGE('',*,*,#10556,.T.);
#13699=ORIENTED_EDGE('',*,*,#10558,.T.);
#13700=ORIENTED_EDGE('',*,*,#10548,.F.);
#13701=ORIENTED_EDGE('',*,*,#10558,.F.);
#13702=ORIENTED_EDGE('',*,*,#10555,.F.);
#13703=ORIENTED_EDGE('',*,*,#10552,.F.);
#13704=ORIENTED_EDGE('',*,*,#10549,.F.);
#13705=ORIENTED_EDGE('',*,*,#10559,.F.);
#13706=ORIENTED_EDGE('',*,*,#10560,.T.);
#13707=ORIENTED_EDGE('',*,*,#10561,.T.);
#13708=ORIENTED_EDGE('',*,*,#10562,.F.);
#13709=ORIENTED_EDGE('',*,*,#10563,.F.);
#13710=ORIENTED_EDGE('',*,*,#10562,.T.);
#13711=ORIENTED_EDGE('',*,*,#10564,.T.);
#13712=ORIENTED_EDGE('',*,*,#10565,.F.);
#13713=ORIENTED_EDGE('',*,*,#10566,.F.);
#13714=ORIENTED_EDGE('',*,*,#10565,.T.);
#13715=ORIENTED_EDGE('',*,*,#10567,.T.);
#13716=ORIENTED_EDGE('',*,*,#10568,.F.);
#13717=ORIENTED_EDGE('',*,*,#10569,.F.);
#13718=ORIENTED_EDGE('',*,*,#10568,.T.);
#13719=ORIENTED_EDGE('',*,*,#10570,.T.);
#13720=ORIENTED_EDGE('',*,*,#10560,.F.);
#13721=ORIENTED_EDGE('',*,*,#10570,.F.);
#13722=ORIENTED_EDGE('',*,*,#10567,.F.);
#13723=ORIENTED_EDGE('',*,*,#10564,.F.);
#13724=ORIENTED_EDGE('',*,*,#10561,.F.);
#13725=ORIENTED_EDGE('',*,*,#10571,.F.);
#13726=ORIENTED_EDGE('',*,*,#10572,.T.);
#13727=ORIENTED_EDGE('',*,*,#10573,.T.);
#13728=ORIENTED_EDGE('',*,*,#10574,.F.);
#13729=ORIENTED_EDGE('',*,*,#10575,.F.);
#13730=ORIENTED_EDGE('',*,*,#10574,.T.);
#13731=ORIENTED_EDGE('',*,*,#10576,.T.);
#13732=ORIENTED_EDGE('',*,*,#10577,.F.);
#13733=ORIENTED_EDGE('',*,*,#10578,.F.);
#13734=ORIENTED_EDGE('',*,*,#10577,.T.);
#13735=ORIENTED_EDGE('',*,*,#10579,.T.);
#13736=ORIENTED_EDGE('',*,*,#10580,.F.);
#13737=ORIENTED_EDGE('',*,*,#10581,.F.);
#13738=ORIENTED_EDGE('',*,*,#10580,.T.);
#13739=ORIENTED_EDGE('',*,*,#10582,.T.);
#13740=ORIENTED_EDGE('',*,*,#10572,.F.);
#13741=ORIENTED_EDGE('',*,*,#10582,.F.);
#13742=ORIENTED_EDGE('',*,*,#10579,.F.);
#13743=ORIENTED_EDGE('',*,*,#10576,.F.);
#13744=ORIENTED_EDGE('',*,*,#10573,.F.);
#13745=ORIENTED_EDGE('',*,*,#10583,.F.);
#13746=ORIENTED_EDGE('',*,*,#10584,.T.);
#13747=ORIENTED_EDGE('',*,*,#10585,.T.);
#13748=ORIENTED_EDGE('',*,*,#10586,.F.);
#13749=ORIENTED_EDGE('',*,*,#10587,.F.);
#13750=ORIENTED_EDGE('',*,*,#10586,.T.);
#13751=ORIENTED_EDGE('',*,*,#10588,.T.);
#13752=ORIENTED_EDGE('',*,*,#10589,.F.);
#13753=ORIENTED_EDGE('',*,*,#10590,.F.);
#13754=ORIENTED_EDGE('',*,*,#10589,.T.);
#13755=ORIENTED_EDGE('',*,*,#10591,.T.);
#13756=ORIENTED_EDGE('',*,*,#10592,.F.);
#13757=ORIENTED_EDGE('',*,*,#10593,.F.);
#13758=ORIENTED_EDGE('',*,*,#10592,.T.);
#13759=ORIENTED_EDGE('',*,*,#10594,.T.);
#13760=ORIENTED_EDGE('',*,*,#10584,.F.);
#13761=ORIENTED_EDGE('',*,*,#10594,.F.);
#13762=ORIENTED_EDGE('',*,*,#10591,.F.);
#13763=ORIENTED_EDGE('',*,*,#10588,.F.);
#13764=ORIENTED_EDGE('',*,*,#10585,.F.);
#13765=ORIENTED_EDGE('',*,*,#10595,.F.);
#13766=ORIENTED_EDGE('',*,*,#10596,.T.);
#13767=ORIENTED_EDGE('',*,*,#10597,.T.);
#13768=ORIENTED_EDGE('',*,*,#10598,.F.);
#13769=ORIENTED_EDGE('',*,*,#10599,.F.);
#13770=ORIENTED_EDGE('',*,*,#10598,.T.);
#13771=ORIENTED_EDGE('',*,*,#10600,.T.);
#13772=ORIENTED_EDGE('',*,*,#10601,.F.);
#13773=ORIENTED_EDGE('',*,*,#10602,.F.);
#13774=ORIENTED_EDGE('',*,*,#10601,.T.);
#13775=ORIENTED_EDGE('',*,*,#10603,.T.);
#13776=ORIENTED_EDGE('',*,*,#10604,.F.);
#13777=ORIENTED_EDGE('',*,*,#10605,.F.);
#13778=ORIENTED_EDGE('',*,*,#10604,.T.);
#13779=ORIENTED_EDGE('',*,*,#10606,.T.);
#13780=ORIENTED_EDGE('',*,*,#10596,.F.);
#13781=ORIENTED_EDGE('',*,*,#10606,.F.);
#13782=ORIENTED_EDGE('',*,*,#10603,.F.);
#13783=ORIENTED_EDGE('',*,*,#10600,.F.);
#13784=ORIENTED_EDGE('',*,*,#10597,.F.);
#13785=ORIENTED_EDGE('',*,*,#10607,.F.);
#13786=ORIENTED_EDGE('',*,*,#10608,.T.);
#13787=ORIENTED_EDGE('',*,*,#10609,.F.);
#13788=ORIENTED_EDGE('',*,*,#10608,.F.);
#13789=ORIENTED_EDGE('',*,*,#10610,.F.);
#13790=ORIENTED_EDGE('',*,*,#10611,.T.);
#13791=ORIENTED_EDGE('',*,*,#10612,.F.);
#13792=ORIENTED_EDGE('',*,*,#10611,.F.);
#13793=ORIENTED_EDGE('',*,*,#10613,.T.);
#13794=ORIENTED_EDGE('',*,*,#10614,.T.);
#13795=ORIENTED_EDGE('',*,*,#10615,.F.);
#13796=ORIENTED_EDGE('',*,*,#10616,.F.);
#13797=ORIENTED_EDGE('',*,*,#10617,.T.);
#13798=ORIENTED_EDGE('',*,*,#10616,.T.);
#13799=ORIENTED_EDGE('',*,*,#10618,.F.);
#13800=ORIENTED_EDGE('',*,*,#10619,.F.);
#13801=ORIENTED_EDGE('',*,*,#10609,.T.);
#13802=ORIENTED_EDGE('',*,*,#10612,.T.);
#13803=ORIENTED_EDGE('',*,*,#10620,.T.);
#13804=ORIENTED_EDGE('',*,*,#10619,.T.);
#13805=ORIENTED_EDGE('',*,*,#10621,.F.);
#13806=ORIENTED_EDGE('',*,*,#10622,.F.);
#13807=ORIENTED_EDGE('',*,*,#10623,.T.);
#13808=ORIENTED_EDGE('',*,*,#10622,.T.);
#13809=ORIENTED_EDGE('',*,*,#10624,.F.);
#13810=ORIENTED_EDGE('',*,*,#10614,.F.);
#13811=ORIENTED_EDGE('',*,*,#10326,.T.);
#13812=ORIENTED_EDGE('',*,*,#10329,.T.);
#13813=ORIENTED_EDGE('',*,*,#10319,.T.);
#13814=ORIENTED_EDGE('',*,*,#10323,.T.);
#13815=ORIENTED_EDGE('',*,*,#10350,.T.);
#13816=ORIENTED_EDGE('',*,*,#10353,.T.);
#13817=ORIENTED_EDGE('',*,*,#10343,.T.);
#13818=ORIENTED_EDGE('',*,*,#10347,.T.);
#13819=ORIENTED_EDGE('',*,*,#10374,.T.);
#13820=ORIENTED_EDGE('',*,*,#10377,.T.);
#13821=ORIENTED_EDGE('',*,*,#10367,.T.);
#13822=ORIENTED_EDGE('',*,*,#10371,.T.);
#13823=ORIENTED_EDGE('',*,*,#10398,.T.);
#13824=ORIENTED_EDGE('',*,*,#10401,.T.);
#13825=ORIENTED_EDGE('',*,*,#10391,.T.);
#13826=ORIENTED_EDGE('',*,*,#10395,.T.);
#13827=ORIENTED_EDGE('',*,*,#10422,.T.);
#13828=ORIENTED_EDGE('',*,*,#10425,.T.);
#13829=ORIENTED_EDGE('',*,*,#10415,.T.);
#13830=ORIENTED_EDGE('',*,*,#10419,.T.);
#13831=ORIENTED_EDGE('',*,*,#10446,.T.);
#13832=ORIENTED_EDGE('',*,*,#10449,.T.);
#13833=ORIENTED_EDGE('',*,*,#10439,.T.);
#13834=ORIENTED_EDGE('',*,*,#10443,.T.);
#13835=ORIENTED_EDGE('',*,*,#10470,.T.);
#13836=ORIENTED_EDGE('',*,*,#10473,.T.);
#13837=ORIENTED_EDGE('',*,*,#10463,.T.);
#13838=ORIENTED_EDGE('',*,*,#10467,.T.);
#13839=ORIENTED_EDGE('',*,*,#10494,.T.);
#13840=ORIENTED_EDGE('',*,*,#10497,.T.);
#13841=ORIENTED_EDGE('',*,*,#10487,.T.);
#13842=ORIENTED_EDGE('',*,*,#10491,.T.);
#13843=ORIENTED_EDGE('',*,*,#10518,.T.);
#13844=ORIENTED_EDGE('',*,*,#10521,.T.);
#13845=ORIENTED_EDGE('',*,*,#10511,.T.);
#13846=ORIENTED_EDGE('',*,*,#10515,.T.);
#13847=ORIENTED_EDGE('',*,*,#10542,.T.);
#13848=ORIENTED_EDGE('',*,*,#10545,.T.);
#13849=ORIENTED_EDGE('',*,*,#10535,.T.);
#13850=ORIENTED_EDGE('',*,*,#10539,.T.);
#13851=ORIENTED_EDGE('',*,*,#10554,.T.);
#13852=ORIENTED_EDGE('',*,*,#10557,.T.);
#13853=ORIENTED_EDGE('',*,*,#10547,.T.);
#13854=ORIENTED_EDGE('',*,*,#10551,.T.);
#13855=ORIENTED_EDGE('',*,*,#10566,.T.);
#13856=ORIENTED_EDGE('',*,*,#10569,.T.);
#13857=ORIENTED_EDGE('',*,*,#10559,.T.);
#13858=ORIENTED_EDGE('',*,*,#10563,.T.);
#13859=ORIENTED_EDGE('',*,*,#10578,.T.);
#13860=ORIENTED_EDGE('',*,*,#10581,.T.);
#13861=ORIENTED_EDGE('',*,*,#10571,.T.);
#13862=ORIENTED_EDGE('',*,*,#10575,.T.);
#13863=ORIENTED_EDGE('',*,*,#10590,.T.);
#13864=ORIENTED_EDGE('',*,*,#10593,.T.);
#13865=ORIENTED_EDGE('',*,*,#10583,.T.);
#13866=ORIENTED_EDGE('',*,*,#10587,.T.);
#13867=ORIENTED_EDGE('',*,*,#10602,.T.);
#13868=ORIENTED_EDGE('',*,*,#10605,.T.);
#13869=ORIENTED_EDGE('',*,*,#10595,.T.);
#13870=ORIENTED_EDGE('',*,*,#10599,.T.);
#13871=ORIENTED_EDGE('',*,*,#10607,.T.);
#13872=ORIENTED_EDGE('',*,*,#10610,.T.);
#13873=ORIENTED_EDGE('',*,*,#10530,.T.);
#13874=ORIENTED_EDGE('',*,*,#10533,.T.);
#13875=ORIENTED_EDGE('',*,*,#10523,.T.);
#13876=ORIENTED_EDGE('',*,*,#10527,.T.);
#13877=ORIENTED_EDGE('',*,*,#10506,.T.);
#13878=ORIENTED_EDGE('',*,*,#10509,.T.);
#13879=ORIENTED_EDGE('',*,*,#10499,.T.);
#13880=ORIENTED_EDGE('',*,*,#10503,.T.);
#13881=ORIENTED_EDGE('',*,*,#10482,.T.);
#13882=ORIENTED_EDGE('',*,*,#10485,.T.);
#13883=ORIENTED_EDGE('',*,*,#10475,.T.);
#13884=ORIENTED_EDGE('',*,*,#10479,.T.);
#13885=ORIENTED_EDGE('',*,*,#10458,.T.);
#13886=ORIENTED_EDGE('',*,*,#10461,.T.);
#13887=ORIENTED_EDGE('',*,*,#10451,.T.);
#13888=ORIENTED_EDGE('',*,*,#10455,.T.);
#13889=ORIENTED_EDGE('',*,*,#10434,.T.);
#13890=ORIENTED_EDGE('',*,*,#10437,.T.);
#13891=ORIENTED_EDGE('',*,*,#10427,.T.);
#13892=ORIENTED_EDGE('',*,*,#10431,.T.);
#13893=ORIENTED_EDGE('',*,*,#10410,.T.);
#13894=ORIENTED_EDGE('',*,*,#10413,.T.);
#13895=ORIENTED_EDGE('',*,*,#10403,.T.);
#13896=ORIENTED_EDGE('',*,*,#10407,.T.);
#13897=ORIENTED_EDGE('',*,*,#10386,.T.);
#13898=ORIENTED_EDGE('',*,*,#10389,.T.);
#13899=ORIENTED_EDGE('',*,*,#10379,.T.);
#13900=ORIENTED_EDGE('',*,*,#10383,.T.);
#13901=ORIENTED_EDGE('',*,*,#10362,.T.);
#13902=ORIENTED_EDGE('',*,*,#10365,.T.);
#13903=ORIENTED_EDGE('',*,*,#10355,.T.);
#13904=ORIENTED_EDGE('',*,*,#10359,.T.);
#13905=ORIENTED_EDGE('',*,*,#10338,.T.);
#13906=ORIENTED_EDGE('',*,*,#10341,.T.);
#13907=ORIENTED_EDGE('',*,*,#10331,.T.);
#13908=ORIENTED_EDGE('',*,*,#10335,.T.);
#13909=ORIENTED_EDGE('',*,*,#10314,.T.);
#13910=ORIENTED_EDGE('',*,*,#10317,.T.);
#13911=ORIENTED_EDGE('',*,*,#10307,.T.);
#13912=ORIENTED_EDGE('',*,*,#10311,.T.);
#13913=ORIENTED_EDGE('',*,*,#10624,.T.);
#13914=ORIENTED_EDGE('',*,*,#10621,.T.);
#13915=ORIENTED_EDGE('',*,*,#10618,.T.);
#13916=ORIENTED_EDGE('',*,*,#10615,.T.);
#13917=ORIENTED_EDGE('',*,*,#10623,.F.);
#13918=ORIENTED_EDGE('',*,*,#10613,.F.);
#13919=ORIENTED_EDGE('',*,*,#10617,.F.);
#13920=ORIENTED_EDGE('',*,*,#10620,.F.);
#17215=CYLINDRICAL_SURFACE('',#19908,0.274999999999999);
#17216=CYLINDRICAL_SURFACE('',#19911,0.275);
#17743=ADVANCED_FACE('',(#2419),#1728,.F.);
#17744=ADVANCED_FACE('',(#2420),#1729,.F.);
#17745=ADVANCED_FACE('',(#2421),#1730,.F.);
#17746=ADVANCED_FACE('',(#2422),#1731,.F.);
#17747=ADVANCED_FACE('',(#2423),#1732,.F.);
#17748=ADVANCED_FACE('',(#2424),#1733,.F.);
#17749=ADVANCED_FACE('',(#2425),#1734,.F.);
#17750=ADVANCED_FACE('',(#2426),#1735,.F.);
#17751=ADVANCED_FACE('',(#2427),#1736,.F.);
#17752=ADVANCED_FACE('',(#2428),#1737,.F.);
#17753=ADVANCED_FACE('',(#2429),#1738,.F.);
#17754=ADVANCED_FACE('',(#2430),#1739,.F.);
#17755=ADVANCED_FACE('',(#2431),#1740,.F.);
#17756=ADVANCED_FACE('',(#2432),#1741,.F.);
#17757=ADVANCED_FACE('',(#2433),#1742,.F.);
#17758=ADVANCED_FACE('',(#2434),#1743,.F.);
#17759=ADVANCED_FACE('',(#2435),#1744,.F.);
#17760=ADVANCED_FACE('',(#2436),#1745,.F.);
#17761=ADVANCED_FACE('',(#2437),#1746,.F.);
#17762=ADVANCED_FACE('',(#2438),#1747,.F.);
#17763=ADVANCED_FACE('',(#2439),#1748,.F.);
#17764=ADVANCED_FACE('',(#2440),#1749,.F.);
#17765=ADVANCED_FACE('',(#2441),#1750,.F.);
#17766=ADVANCED_FACE('',(#2442),#1751,.F.);
#17767=ADVANCED_FACE('',(#2443),#1752,.F.);
#17768=ADVANCED_FACE('',(#2444),#1753,.F.);
#17769=ADVANCED_FACE('',(#2445),#1754,.F.);
#17770=ADVANCED_FACE('',(#2446),#1755,.F.);
#17771=ADVANCED_FACE('',(#2447),#1756,.F.);
#17772=ADVANCED_FACE('',(#2448),#1757,.F.);
#17773=ADVANCED_FACE('',(#2449),#1758,.F.);
#17774=ADVANCED_FACE('',(#2450),#1759,.F.);
#17775=ADVANCED_FACE('',(#2451),#1760,.F.);
#17776=ADVANCED_FACE('',(#2452),#1761,.F.);
#17777=ADVANCED_FACE('',(#2453),#1762,.F.);
#17778=ADVANCED_FACE('',(#2454),#1763,.F.);
#17779=ADVANCED_FACE('',(#2455),#1764,.F.);
#17780=ADVANCED_FACE('',(#2456),#1765,.F.);
#17781=ADVANCED_FACE('',(#2457),#1766,.F.);
#17782=ADVANCED_FACE('',(#2458),#1767,.F.);
#17783=ADVANCED_FACE('',(#2459),#1768,.F.);
#17784=ADVANCED_FACE('',(#2460),#1769,.F.);
#17785=ADVANCED_FACE('',(#2461),#1770,.F.);
#17786=ADVANCED_FACE('',(#2462),#1771,.F.);
#17787=ADVANCED_FACE('',(#2463),#1772,.F.);
#17788=ADVANCED_FACE('',(#2464),#1773,.F.);
#17789=ADVANCED_FACE('',(#2465),#1774,.F.);
#17790=ADVANCED_FACE('',(#2466),#1775,.F.);
#17791=ADVANCED_FACE('',(#2467),#1776,.F.);
#17792=ADVANCED_FACE('',(#2468),#1777,.F.);
#17793=ADVANCED_FACE('',(#2469),#1778,.F.);
#17794=ADVANCED_FACE('',(#2470),#1779,.F.);
#17795=ADVANCED_FACE('',(#2471),#1780,.F.);
#17796=ADVANCED_FACE('',(#2472),#1781,.F.);
#17797=ADVANCED_FACE('',(#2473),#1782,.F.);
#17798=ADVANCED_FACE('',(#2474),#1783,.F.);
#17799=ADVANCED_FACE('',(#2475),#1784,.F.);
#17800=ADVANCED_FACE('',(#2476),#1785,.F.);
#17801=ADVANCED_FACE('',(#2477),#1786,.F.);
#17802=ADVANCED_FACE('',(#2478),#1787,.F.);
#17803=ADVANCED_FACE('',(#2479),#1788,.F.);
#17804=ADVANCED_FACE('',(#2480),#1789,.F.);
#17805=ADVANCED_FACE('',(#2481),#1790,.F.);
#17806=ADVANCED_FACE('',(#2482),#1791,.F.);
#17807=ADVANCED_FACE('',(#2483),#1792,.F.);
#17808=ADVANCED_FACE('',(#2484),#1793,.F.);
#17809=ADVANCED_FACE('',(#2485),#1794,.F.);
#17810=ADVANCED_FACE('',(#2486),#1795,.F.);
#17811=ADVANCED_FACE('',(#2487),#1796,.F.);
#17812=ADVANCED_FACE('',(#2488),#1797,.F.);
#17813=ADVANCED_FACE('',(#2489),#1798,.F.);
#17814=ADVANCED_FACE('',(#2490),#1799,.F.);
#17815=ADVANCED_FACE('',(#2491),#1800,.F.);
#17816=ADVANCED_FACE('',(#2492),#1801,.F.);
#17817=ADVANCED_FACE('',(#2493),#1802,.F.);
#17818=ADVANCED_FACE('',(#2494),#1803,.F.);
#17819=ADVANCED_FACE('',(#2495),#1804,.F.);
#17820=ADVANCED_FACE('',(#2496),#1805,.F.);
#17821=ADVANCED_FACE('',(#2497),#1806,.F.);
#17822=ADVANCED_FACE('',(#2498),#1807,.F.);
#17823=ADVANCED_FACE('',(#2499),#1808,.F.);
#17824=ADVANCED_FACE('',(#2500),#1809,.F.);
#17825=ADVANCED_FACE('',(#2501),#1810,.F.);
#17826=ADVANCED_FACE('',(#2502),#1811,.F.);
#17827=ADVANCED_FACE('',(#2503),#1812,.F.);
#17828=ADVANCED_FACE('',(#2504),#1813,.F.);
#17829=ADVANCED_FACE('',(#2505),#1814,.F.);
#17830=ADVANCED_FACE('',(#2506),#1815,.F.);
#17831=ADVANCED_FACE('',(#2507),#1816,.F.);
#17832=ADVANCED_FACE('',(#2508),#1817,.F.);
#17833=ADVANCED_FACE('',(#2509),#1818,.F.);
#17834=ADVANCED_FACE('',(#2510),#1819,.F.);
#17835=ADVANCED_FACE('',(#2511),#1820,.F.);
#17836=ADVANCED_FACE('',(#2512),#1821,.F.);
#17837=ADVANCED_FACE('',(#2513),#1822,.F.);
#17838=ADVANCED_FACE('',(#2514),#1823,.F.);
#17839=ADVANCED_FACE('',(#2515),#1824,.F.);
#17840=ADVANCED_FACE('',(#2516),#1825,.F.);
#17841=ADVANCED_FACE('',(#2517),#1826,.F.);
#17842=ADVANCED_FACE('',(#2518),#1827,.F.);
#17843=ADVANCED_FACE('',(#2519),#1828,.F.);
#17844=ADVANCED_FACE('',(#2520),#1829,.F.);
#17845=ADVANCED_FACE('',(#2521),#1830,.F.);
#17846=ADVANCED_FACE('',(#2522),#1831,.F.);
#17847=ADVANCED_FACE('',(#2523),#1832,.F.);
#17848=ADVANCED_FACE('',(#2524),#1833,.F.);
#17849=ADVANCED_FACE('',(#2525),#1834,.F.);
#17850=ADVANCED_FACE('',(#2526),#1835,.F.);
#17851=ADVANCED_FACE('',(#2527),#1836,.F.);
#17852=ADVANCED_FACE('',(#2528),#1837,.F.);
#17853=ADVANCED_FACE('',(#2529),#1838,.F.);
#17854=ADVANCED_FACE('',(#2530),#1839,.F.);
#17855=ADVANCED_FACE('',(#2531),#1840,.F.);
#17856=ADVANCED_FACE('',(#2532),#1841,.F.);
#17857=ADVANCED_FACE('',(#2533),#1842,.F.);
#17858=ADVANCED_FACE('',(#2534),#1843,.F.);
#17859=ADVANCED_FACE('',(#2535),#1844,.F.);
#17860=ADVANCED_FACE('',(#2536),#1845,.F.);
#17861=ADVANCED_FACE('',(#2537),#1846,.F.);
#17862=ADVANCED_FACE('',(#2538),#1847,.F.);
#17863=ADVANCED_FACE('',(#2539),#1848,.F.);
#17864=ADVANCED_FACE('',(#2540),#1849,.F.);
#17865=ADVANCED_FACE('',(#2541),#1850,.F.);
#17866=ADVANCED_FACE('',(#2542),#1851,.F.);
#17867=ADVANCED_FACE('',(#2543),#1852,.F.);
#17868=ADVANCED_FACE('',(#2544),#17215,.F.);
#17869=ADVANCED_FACE('',(#2545),#17216,.F.);
#17870=ADVANCED_FACE('',(#2546),#1853,.T.);
#17871=ADVANCED_FACE('',(#2547,#1410,#1411),#1854,.T.);
#17872=ADVANCED_FACE('',(#2548),#1855,.T.);
#17873=ADVANCED_FACE('',(#2549,#1412,#1413,#1414,#1415,#1416,#1417,#1418,
#1419,#1420,#1421,#1422,#1423,#1424,#1425,#1426,#1427,#1428,#1429,#1430,
#1431,#1432,#1433,#1434,#1435,#1436,#1437,#1438),#1856,.T.);
#17874=ADVANCED_FACE('',(#2550),#1857,.T.);
#17875=ADVANCED_FACE('',(#2551),#1858,.F.);
#18560=CLOSED_SHELL('',(#17743,#17744,#17745,#17746,#17747,#17748,#17749,
#17750,#17751,#17752,#17753,#17754,#17755,#17756,#17757,#17758,#17759,#17760,
#17761,#17762,#17763,#17764,#17765,#17766,#17767,#17768,#17769,#17770,#17771,
#17772,#17773,#17774,#17775,#17776,#17777,#17778,#17779,#17780,#17781,#17782,
#17783,#17784,#17785,#17786,#17787,#17788,#17789,#17790,#17791,#17792,#17793,
#17794,#17795,#17796,#17797,#17798,#17799,#17800,#17801,#17802,#17803,#17804,
#17805,#17806,#17807,#17808,#17809,#17810,#17811,#17812,#17813,#17814,#17815,
#17816,#17817,#17818,#17819,#17820,#17821,#17822,#17823,#17824,#17825,#17826,
#17827,#17828,#17829,#17830,#17831,#17832,#17833,#17834,#17835,#17836,#17837,
#17838,#17839,#17840,#17841,#17842,#17843,#17844,#17845,#17846,#17847,#17848,
#17849,#17850,#17851,#17852,#17853,#17854,#17855,#17856,#17857,#17858,#17859,
#17860,#17861,#17862,#17863,#17864,#17865,#17866,#17867,#17868,#17869,#17870,
#17871,#17872,#17873,#17874,#17875));
#19782=AXIS2_PLACEMENT_3D('',#27612,#22498,#22499);
#19783=AXIS2_PLACEMENT_3D('',#27613,#22500,#22501);
#19784=AXIS2_PLACEMENT_3D('',#27622,#22506,#22507);
#19785=AXIS2_PLACEMENT_3D('',#27628,#22511,#22512);
#19786=AXIS2_PLACEMENT_3D('',#27634,#22516,#22517);
#19787=AXIS2_PLACEMENT_3D('',#27637,#22520,#22521);
#19788=AXIS2_PLACEMENT_3D('',#27638,#22522,#22523);
#19789=AXIS2_PLACEMENT_3D('',#27647,#22528,#22529);
#19790=AXIS2_PLACEMENT_3D('',#27653,#22533,#22534);
#19791=AXIS2_PLACEMENT_3D('',#27659,#22538,#22539);
#19792=AXIS2_PLACEMENT_3D('',#27662,#22542,#22543);
#19793=AXIS2_PLACEMENT_3D('',#27663,#22544,#22545);
#19794=AXIS2_PLACEMENT_3D('',#27672,#22550,#22551);
#19795=AXIS2_PLACEMENT_3D('',#27678,#22555,#22556);
#19796=AXIS2_PLACEMENT_3D('',#27684,#22560,#22561);
#19797=AXIS2_PLACEMENT_3D('',#27687,#22564,#22565);
#19798=AXIS2_PLACEMENT_3D('',#27688,#22566,#22567);
#19799=AXIS2_PLACEMENT_3D('',#27697,#22572,#22573);
#19800=AXIS2_PLACEMENT_3D('',#27703,#22577,#22578);
#19801=AXIS2_PLACEMENT_3D('',#27709,#22582,#22583);
#19802=AXIS2_PLACEMENT_3D('',#27712,#22586,#22587);
#19803=AXIS2_PLACEMENT_3D('',#27713,#22588,#22589);
#19804=AXIS2_PLACEMENT_3D('',#27722,#22594,#22595);
#19805=AXIS2_PLACEMENT_3D('',#27728,#22599,#22600);
#19806=AXIS2_PLACEMENT_3D('',#27734,#22604,#22605);
#19807=AXIS2_PLACEMENT_3D('',#27737,#22608,#22609);
#19808=AXIS2_PLACEMENT_3D('',#27738,#22610,#22611);
#19809=AXIS2_PLACEMENT_3D('',#27747,#22616,#22617);
#19810=AXIS2_PLACEMENT_3D('',#27753,#22621,#22622);
#19811=AXIS2_PLACEMENT_3D('',#27759,#22626,#22627);
#19812=AXIS2_PLACEMENT_3D('',#27762,#22630,#22631);
#19813=AXIS2_PLACEMENT_3D('',#27763,#22632,#22633);
#19814=AXIS2_PLACEMENT_3D('',#27772,#22638,#22639);
#19815=AXIS2_PLACEMENT_3D('',#27778,#22643,#22644);
#19816=AXIS2_PLACEMENT_3D('',#27784,#22648,#22649);
#19817=AXIS2_PLACEMENT_3D('',#27787,#22652,#22653);
#19818=AXIS2_PLACEMENT_3D('',#27788,#22654,#22655);
#19819=AXIS2_PLACEMENT_3D('',#27797,#22660,#22661);
#19820=AXIS2_PLACEMENT_3D('',#27803,#22665,#22666);
#19821=AXIS2_PLACEMENT_3D('',#27809,#22670,#22671);
#19822=AXIS2_PLACEMENT_3D('',#27812,#22674,#22675);
#19823=AXIS2_PLACEMENT_3D('',#27813,#22676,#22677);
#19824=AXIS2_PLACEMENT_3D('',#27822,#22682,#22683);
#19825=AXIS2_PLACEMENT_3D('',#27828,#22687,#22688);
#19826=AXIS2_PLACEMENT_3D('',#27834,#22692,#22693);
#19827=AXIS2_PLACEMENT_3D('',#27837,#22696,#22697);
#19828=AXIS2_PLACEMENT_3D('',#27838,#22698,#22699);
#19829=AXIS2_PLACEMENT_3D('',#27847,#22704,#22705);
#19830=AXIS2_PLACEMENT_3D('',#27853,#22709,#22710);
#19831=AXIS2_PLACEMENT_3D('',#27859,#22714,#22715);
#19832=AXIS2_PLACEMENT_3D('',#27862,#22718,#22719);
#19833=AXIS2_PLACEMENT_3D('',#27863,#22720,#22721);
#19834=AXIS2_PLACEMENT_3D('',#27872,#22726,#22727);
#19835=AXIS2_PLACEMENT_3D('',#27878,#22731,#22732);
#19836=AXIS2_PLACEMENT_3D('',#27884,#22736,#22737);
#19837=AXIS2_PLACEMENT_3D('',#27887,#22740,#22741);
#19838=AXIS2_PLACEMENT_3D('',#27888,#22742,#22743);
#19839=AXIS2_PLACEMENT_3D('',#27897,#22748,#22749);
#19840=AXIS2_PLACEMENT_3D('',#27903,#22753,#22754);
#19841=AXIS2_PLACEMENT_3D('',#27909,#22758,#22759);
#19842=AXIS2_PLACEMENT_3D('',#27912,#22762,#22763);
#19843=AXIS2_PLACEMENT_3D('',#27913,#22764,#22765);
#19844=AXIS2_PLACEMENT_3D('',#27922,#22770,#22771);
#19845=AXIS2_PLACEMENT_3D('',#27928,#22775,#22776);
#19846=AXIS2_PLACEMENT_3D('',#27934,#22780,#22781);
#19847=AXIS2_PLACEMENT_3D('',#27937,#22784,#22785);
#19848=AXIS2_PLACEMENT_3D('',#27938,#22786,#22787);
#19849=AXIS2_PLACEMENT_3D('',#27947,#22792,#22793);
#19850=AXIS2_PLACEMENT_3D('',#27953,#22797,#22798);
#19851=AXIS2_PLACEMENT_3D('',#27959,#22802,#22803);
#19852=AXIS2_PLACEMENT_3D('',#27962,#22806,#22807);
#19853=AXIS2_PLACEMENT_3D('',#27963,#22808,#22809);
#19854=AXIS2_PLACEMENT_3D('',#27972,#22814,#22815);
#19855=AXIS2_PLACEMENT_3D('',#27978,#22819,#22820);
#19856=AXIS2_PLACEMENT_3D('',#27984,#22824,#22825);
#19857=AXIS2_PLACEMENT_3D('',#27987,#22828,#22829);
#19858=AXIS2_PLACEMENT_3D('',#27988,#22830,#22831);
#19859=AXIS2_PLACEMENT_3D('',#27997,#22836,#22837);
#19860=AXIS2_PLACEMENT_3D('',#28003,#22841,#22842);
#19861=AXIS2_PLACEMENT_3D('',#28009,#22846,#22847);
#19862=AXIS2_PLACEMENT_3D('',#28012,#22850,#22851);
#19863=AXIS2_PLACEMENT_3D('',#28013,#22852,#22853);
#19864=AXIS2_PLACEMENT_3D('',#28022,#22858,#22859);
#19865=AXIS2_PLACEMENT_3D('',#28028,#22863,#22864);
#19866=AXIS2_PLACEMENT_3D('',#28034,#22868,#22869);
#19867=AXIS2_PLACEMENT_3D('',#28037,#22872,#22873);
#19868=AXIS2_PLACEMENT_3D('',#28038,#22874,#22875);
#19869=AXIS2_PLACEMENT_3D('',#28047,#22880,#22881);
#19870=AXIS2_PLACEMENT_3D('',#28053,#22885,#22886);
#19871=AXIS2_PLACEMENT_3D('',#28059,#22890,#22891);
#19872=AXIS2_PLACEMENT_3D('',#28062,#22894,#22895);
#19873=AXIS2_PLACEMENT_3D('',#28063,#22896,#22897);
#19874=AXIS2_PLACEMENT_3D('',#28072,#22902,#22903);
#19875=AXIS2_PLACEMENT_3D('',#28078,#22907,#22908);
#19876=AXIS2_PLACEMENT_3D('',#28084,#22912,#22913);
#19877=AXIS2_PLACEMENT_3D('',#28087,#22916,#22917);
#19878=AXIS2_PLACEMENT_3D('',#28088,#22918,#22919);
#19879=AXIS2_PLACEMENT_3D('',#28097,#22924,#22925);
#19880=AXIS2_PLACEMENT_3D('',#28103,#22929,#22930);
#19881=AXIS2_PLACEMENT_3D('',#28109,#22934,#22935);
#19882=AXIS2_PLACEMENT_3D('',#28112,#22938,#22939);
#19883=AXIS2_PLACEMENT_3D('',#28113,#22940,#22941);
#19884=AXIS2_PLACEMENT_3D('',#28122,#22946,#22947);
#19885=AXIS2_PLACEMENT_3D('',#28128,#22951,#22952);
#19886=AXIS2_PLACEMENT_3D('',#28134,#22956,#22957);
#19887=AXIS2_PLACEMENT_3D('',#28137,#22960,#22961);
#19888=AXIS2_PLACEMENT_3D('',#28138,#22962,#22963);
#19889=AXIS2_PLACEMENT_3D('',#28147,#22968,#22969);
#19890=AXIS2_PLACEMENT_3D('',#28153,#22973,#22974);
#19891=AXIS2_PLACEMENT_3D('',#28159,#22978,#22979);
#19892=AXIS2_PLACEMENT_3D('',#28162,#22982,#22983);
#19893=AXIS2_PLACEMENT_3D('',#28163,#22984,#22985);
#19894=AXIS2_PLACEMENT_3D('',#28172,#22990,#22991);
#19895=AXIS2_PLACEMENT_3D('',#28178,#22995,#22996);
#19896=AXIS2_PLACEMENT_3D('',#28184,#23000,#23001);
#19897=AXIS2_PLACEMENT_3D('',#28187,#23004,#23005);
#19898=AXIS2_PLACEMENT_3D('',#28188,#23006,#23007);
#19899=AXIS2_PLACEMENT_3D('',#28197,#23012,#23013);
#19900=AXIS2_PLACEMENT_3D('',#28203,#23017,#23018);
#19901=AXIS2_PLACEMENT_3D('',#28209,#23022,#23023);
#19902=AXIS2_PLACEMENT_3D('',#28212,#23026,#23027);
#19903=AXIS2_PLACEMENT_3D('',#28213,#23028,#23029);
#19904=AXIS2_PLACEMENT_3D('',#28222,#23034,#23035);
#19905=AXIS2_PLACEMENT_3D('',#28228,#23039,#23040);
#19906=AXIS2_PLACEMENT_3D('',#28234,#23044,#23045);
#19907=AXIS2_PLACEMENT_3D('',#28237,#23048,#23049);
#19908=AXIS2_PLACEMENT_3D('',#28238,#23050,#23051);
#19909=AXIS2_PLACEMENT_3D('',#28240,#23052,#23053);
#19910=AXIS2_PLACEMENT_3D('',#28243,#23055,#23056);
#19911=AXIS2_PLACEMENT_3D('',#28244,#23057,#23058);
#19912=AXIS2_PLACEMENT_3D('',#28246,#23059,#23060);
#19913=AXIS2_PLACEMENT_3D('',#28249,#23062,#23063);
#19914=AXIS2_PLACEMENT_3D('',#28250,#23064,#23065);
#19915=AXIS2_PLACEMENT_3D('',#28259,#23070,#23071);
#19916=AXIS2_PLACEMENT_3D('',#28265,#23075,#23076);
#19917=AXIS2_PLACEMENT_3D('',#28271,#23080,#23081);
#19918=AXIS2_PLACEMENT_3D('',#28274,#23084,#23085);
#19919=AXIS2_PLACEMENT_3D('',#28275,#23086,#23087);
#22498=DIRECTION('axis',(0.,0.,1.));
#22499=DIRECTION('refdir',(1.,0.,0.));
#22500=DIRECTION('center_axis',(0.,0.,-1.));
#22501=DIRECTION('ref_axis',(0.,1.,0.));
#22502=DIRECTION('',(0.,1.,0.));
#22503=DIRECTION('',(1.,0.,0.));
#22504=DIRECTION('',(0.,1.,0.));
#22505=DIRECTION('',(1.,0.,0.));
#22506=DIRECTION('center_axis',(0.,1.,0.));
#22507=DIRECTION('ref_axis',(0.,0.,1.));
#22508=DIRECTION('',(0.,0.,1.));
#22509=DIRECTION('',(0.,0.,1.));
#22510=DIRECTION('',(1.,0.,0.));
#22511=DIRECTION('center_axis',(0.,0.,1.));
#22512=DIRECTION('ref_axis',(0.,-1.,0.));
#22513=DIRECTION('',(0.,-1.,0.));
#22514=DIRECTION('',(0.,-1.,0.));
#22515=DIRECTION('',(1.,0.,0.));
#22516=DIRECTION('center_axis',(0.,-1.,0.));
#22517=DIRECTION('ref_axis',(0.,0.,-1.));
#22518=DIRECTION('',(0.,0.,-1.));
#22519=DIRECTION('',(0.,0.,-1.));
#22520=DIRECTION('center_axis',(1.,0.,0.));
#22521=DIRECTION('ref_axis',(0.,0.,-1.));
#22522=DIRECTION('center_axis',(0.,0.,-1.));
#22523=DIRECTION('ref_axis',(0.,1.,0.));
#22524=DIRECTION('',(0.,1.,0.));
#22525=DIRECTION('',(1.,0.,0.));
#22526=DIRECTION('',(0.,1.,0.));
#22527=DIRECTION('',(1.,0.,0.));
#22528=DIRECTION('center_axis',(0.,1.,0.));
#22529=DIRECTION('ref_axis',(0.,0.,1.));
#22530=DIRECTION('',(0.,0.,1.));
#22531=DIRECTION('',(0.,0.,1.));
#22532=DIRECTION('',(1.,0.,0.));
#22533=DIRECTION('center_axis',(0.,0.,1.));
#22534=DIRECTION('ref_axis',(0.,-1.,0.));
#22535=DIRECTION('',(0.,-1.,0.));
#22536=DIRECTION('',(0.,-1.,0.));
#22537=DIRECTION('',(1.,0.,0.));
#22538=DIRECTION('center_axis',(0.,-1.,0.));
#22539=DIRECTION('ref_axis',(0.,0.,-1.));
#22540=DIRECTION('',(0.,0.,-1.));
#22541=DIRECTION('',(0.,0.,-1.));
#22542=DIRECTION('center_axis',(1.,0.,0.));
#22543=DIRECTION('ref_axis',(0.,0.,-1.));
#22544=DIRECTION('center_axis',(0.,0.,-1.));
#22545=DIRECTION('ref_axis',(0.,1.,0.));
#22546=DIRECTION('',(0.,1.,0.));
#22547=DIRECTION('',(1.,0.,0.));
#22548=DIRECTION('',(0.,1.,0.));
#22549=DIRECTION('',(1.,0.,0.));
#22550=DIRECTION('center_axis',(0.,1.,0.));
#22551=DIRECTION('ref_axis',(0.,0.,1.));
#22552=DIRECTION('',(0.,0.,1.));
#22553=DIRECTION('',(0.,0.,1.));
#22554=DIRECTION('',(1.,0.,0.));
#22555=DIRECTION('center_axis',(0.,0.,1.));
#22556=DIRECTION('ref_axis',(0.,-1.,0.));
#22557=DIRECTION('',(0.,-1.,0.));
#22558=DIRECTION('',(0.,-1.,0.));
#22559=DIRECTION('',(1.,0.,0.));
#22560=DIRECTION('center_axis',(0.,-1.,0.));
#22561=DIRECTION('ref_axis',(0.,0.,-1.));
#22562=DIRECTION('',(0.,0.,-1.));
#22563=DIRECTION('',(0.,0.,-1.));
#22564=DIRECTION('center_axis',(1.,0.,0.));
#22565=DIRECTION('ref_axis',(0.,0.,-1.));
#22566=DIRECTION('center_axis',(0.,0.,-1.));
#22567=DIRECTION('ref_axis',(0.,1.,0.));
#22568=DIRECTION('',(0.,1.,0.));
#22569=DIRECTION('',(1.,0.,0.));
#22570=DIRECTION('',(0.,1.,0.));
#22571=DIRECTION('',(1.,0.,0.));
#22572=DIRECTION('center_axis',(0.,1.,0.));
#22573=DIRECTION('ref_axis',(0.,0.,1.));
#22574=DIRECTION('',(0.,0.,1.));
#22575=DIRECTION('',(0.,0.,1.));
#22576=DIRECTION('',(1.,0.,0.));
#22577=DIRECTION('center_axis',(0.,0.,1.));
#22578=DIRECTION('ref_axis',(0.,-1.,0.));
#22579=DIRECTION('',(0.,-1.,0.));
#22580=DIRECTION('',(0.,-1.,0.));
#22581=DIRECTION('',(1.,0.,0.));
#22582=DIRECTION('center_axis',(0.,-1.,0.));
#22583=DIRECTION('ref_axis',(0.,0.,-1.));
#22584=DIRECTION('',(0.,0.,-1.));
#22585=DIRECTION('',(0.,0.,-1.));
#22586=DIRECTION('center_axis',(1.,0.,0.));
#22587=DIRECTION('ref_axis',(0.,0.,-1.));
#22588=DIRECTION('center_axis',(0.,0.,-1.));
#22589=DIRECTION('ref_axis',(0.,1.,0.));
#22590=DIRECTION('',(0.,1.,0.));
#22591=DIRECTION('',(1.,0.,0.));
#22592=DIRECTION('',(0.,1.,0.));
#22593=DIRECTION('',(1.,0.,0.));
#22594=DIRECTION('center_axis',(0.,1.,0.));
#22595=DIRECTION('ref_axis',(0.,0.,1.));
#22596=DIRECTION('',(0.,0.,1.));
#22597=DIRECTION('',(0.,0.,1.));
#22598=DIRECTION('',(1.,0.,0.));
#22599=DIRECTION('center_axis',(0.,0.,1.));
#22600=DIRECTION('ref_axis',(0.,-1.,0.));
#22601=DIRECTION('',(0.,-1.,0.));
#22602=DIRECTION('',(0.,-1.,0.));
#22603=DIRECTION('',(1.,0.,0.));
#22604=DIRECTION('center_axis',(0.,-1.,0.));
#22605=DIRECTION('ref_axis',(0.,0.,-1.));
#22606=DIRECTION('',(0.,0.,-1.));
#22607=DIRECTION('',(0.,0.,-1.));
#22608=DIRECTION('center_axis',(1.,0.,0.));
#22609=DIRECTION('ref_axis',(0.,0.,-1.));
#22610=DIRECTION('center_axis',(0.,0.,-1.));
#22611=DIRECTION('ref_axis',(0.,1.,0.));
#22612=DIRECTION('',(0.,1.,0.));
#22613=DIRECTION('',(1.,0.,0.));
#22614=DIRECTION('',(0.,1.,0.));
#22615=DIRECTION('',(1.,0.,0.));
#22616=DIRECTION('center_axis',(0.,1.,0.));
#22617=DIRECTION('ref_axis',(0.,0.,1.));
#22618=DIRECTION('',(0.,0.,1.));
#22619=DIRECTION('',(0.,0.,1.));
#22620=DIRECTION('',(1.,0.,0.));
#22621=DIRECTION('center_axis',(0.,0.,1.));
#22622=DIRECTION('ref_axis',(0.,-1.,0.));
#22623=DIRECTION('',(0.,-1.,0.));
#22624=DIRECTION('',(0.,-1.,0.));
#22625=DIRECTION('',(1.,0.,0.));
#22626=DIRECTION('center_axis',(0.,-1.,0.));
#22627=DIRECTION('ref_axis',(0.,0.,-1.));
#22628=DIRECTION('',(0.,0.,-1.));
#22629=DIRECTION('',(0.,0.,-1.));
#22630=DIRECTION('center_axis',(1.,0.,0.));
#22631=DIRECTION('ref_axis',(0.,0.,-1.));
#22632=DIRECTION('center_axis',(0.,0.,-1.));
#22633=DIRECTION('ref_axis',(0.,1.,0.));
#22634=DIRECTION('',(0.,1.,0.));
#22635=DIRECTION('',(1.,0.,0.));
#22636=DIRECTION('',(0.,1.,0.));
#22637=DIRECTION('',(1.,0.,0.));
#22638=DIRECTION('center_axis',(0.,1.,0.));
#22639=DIRECTION('ref_axis',(0.,0.,1.));
#22640=DIRECTION('',(0.,0.,1.));
#22641=DIRECTION('',(0.,0.,1.));
#22642=DIRECTION('',(1.,0.,0.));
#22643=DIRECTION('center_axis',(0.,0.,1.));
#22644=DIRECTION('ref_axis',(0.,-1.,0.));
#22645=DIRECTION('',(0.,-1.,0.));
#22646=DIRECTION('',(0.,-1.,0.));
#22647=DIRECTION('',(1.,0.,0.));
#22648=DIRECTION('center_axis',(0.,-1.,0.));
#22649=DIRECTION('ref_axis',(0.,0.,-1.));
#22650=DIRECTION('',(0.,0.,-1.));
#22651=DIRECTION('',(0.,0.,-1.));
#22652=DIRECTION('center_axis',(1.,0.,0.));
#22653=DIRECTION('ref_axis',(0.,0.,-1.));
#22654=DIRECTION('center_axis',(0.,0.,-1.));
#22655=DIRECTION('ref_axis',(0.,1.,0.));
#22656=DIRECTION('',(0.,1.,0.));
#22657=DIRECTION('',(1.,0.,0.));
#22658=DIRECTION('',(0.,1.,0.));
#22659=DIRECTION('',(1.,0.,0.));
#22660=DIRECTION('center_axis',(0.,1.,0.));
#22661=DIRECTION('ref_axis',(0.,0.,1.));
#22662=DIRECTION('',(0.,0.,1.));
#22663=DIRECTION('',(0.,0.,1.));
#22664=DIRECTION('',(1.,0.,0.));
#22665=DIRECTION('center_axis',(0.,0.,1.));
#22666=DIRECTION('ref_axis',(0.,-1.,0.));
#22667=DIRECTION('',(0.,-1.,0.));
#22668=DIRECTION('',(0.,-1.,0.));
#22669=DIRECTION('',(1.,0.,0.));
#22670=DIRECTION('center_axis',(0.,-1.,0.));
#22671=DIRECTION('ref_axis',(0.,0.,-1.));
#22672=DIRECTION('',(0.,0.,-1.));
#22673=DIRECTION('',(0.,0.,-1.));
#22674=DIRECTION('center_axis',(1.,0.,0.));
#22675=DIRECTION('ref_axis',(0.,0.,-1.));
#22676=DIRECTION('center_axis',(0.,0.,-1.));
#22677=DIRECTION('ref_axis',(0.,1.,0.));
#22678=DIRECTION('',(0.,1.,0.));
#22679=DIRECTION('',(1.,0.,0.));
#22680=DIRECTION('',(0.,1.,0.));
#22681=DIRECTION('',(1.,0.,0.));
#22682=DIRECTION('center_axis',(0.,1.,0.));
#22683=DIRECTION('ref_axis',(0.,0.,1.));
#22684=DIRECTION('',(0.,0.,1.));
#22685=DIRECTION('',(0.,0.,1.));
#22686=DIRECTION('',(1.,0.,0.));
#22687=DIRECTION('center_axis',(0.,0.,1.));
#22688=DIRECTION('ref_axis',(0.,-1.,0.));
#22689=DIRECTION('',(0.,-1.,0.));
#22690=DIRECTION('',(0.,-1.,0.));
#22691=DIRECTION('',(1.,0.,0.));
#22692=DIRECTION('center_axis',(0.,-1.,0.));
#22693=DIRECTION('ref_axis',(0.,0.,-1.));
#22694=DIRECTION('',(0.,0.,-1.));
#22695=DIRECTION('',(0.,0.,-1.));
#22696=DIRECTION('center_axis',(1.,0.,0.));
#22697=DIRECTION('ref_axis',(0.,0.,-1.));
#22698=DIRECTION('center_axis',(0.,0.,-1.));
#22699=DIRECTION('ref_axis',(0.,1.,0.));
#22700=DIRECTION('',(0.,1.,0.));
#22701=DIRECTION('',(1.,0.,0.));
#22702=DIRECTION('',(0.,1.,0.));
#22703=DIRECTION('',(1.,0.,0.));
#22704=DIRECTION('center_axis',(0.,1.,0.));
#22705=DIRECTION('ref_axis',(0.,0.,1.));
#22706=DIRECTION('',(0.,0.,1.));
#22707=DIRECTION('',(0.,0.,1.));
#22708=DIRECTION('',(1.,0.,0.));
#22709=DIRECTION('center_axis',(0.,0.,1.));
#22710=DIRECTION('ref_axis',(0.,-1.,0.));
#22711=DIRECTION('',(0.,-1.,0.));
#22712=DIRECTION('',(0.,-1.,0.));
#22713=DIRECTION('',(1.,0.,0.));
#22714=DIRECTION('center_axis',(0.,-1.,0.));
#22715=DIRECTION('ref_axis',(0.,0.,-1.));
#22716=DIRECTION('',(0.,0.,-1.));
#22717=DIRECTION('',(0.,0.,-1.));
#22718=DIRECTION('center_axis',(1.,0.,0.));
#22719=DIRECTION('ref_axis',(0.,0.,-1.));
#22720=DIRECTION('center_axis',(0.,0.,-1.));
#22721=DIRECTION('ref_axis',(0.,1.,0.));
#22722=DIRECTION('',(0.,1.,0.));
#22723=DIRECTION('',(1.,0.,0.));
#22724=DIRECTION('',(0.,1.,0.));
#22725=DIRECTION('',(1.,0.,0.));
#22726=DIRECTION('center_axis',(0.,1.,0.));
#22727=DIRECTION('ref_axis',(0.,0.,1.));
#22728=DIRECTION('',(0.,0.,1.));
#22729=DIRECTION('',(0.,0.,1.));
#22730=DIRECTION('',(1.,0.,0.));
#22731=DIRECTION('center_axis',(0.,0.,1.));
#22732=DIRECTION('ref_axis',(0.,-1.,0.));
#22733=DIRECTION('',(0.,-1.,0.));
#22734=DIRECTION('',(0.,-1.,0.));
#22735=DIRECTION('',(1.,0.,0.));
#22736=DIRECTION('center_axis',(0.,-1.,0.));
#22737=DIRECTION('ref_axis',(0.,0.,-1.));
#22738=DIRECTION('',(0.,0.,-1.));
#22739=DIRECTION('',(0.,0.,-1.));
#22740=DIRECTION('center_axis',(1.,0.,0.));
#22741=DIRECTION('ref_axis',(0.,0.,-1.));
#22742=DIRECTION('center_axis',(0.,0.,-1.));
#22743=DIRECTION('ref_axis',(0.,1.,0.));
#22744=DIRECTION('',(0.,1.,0.));
#22745=DIRECTION('',(1.,0.,0.));
#22746=DIRECTION('',(0.,1.,0.));
#22747=DIRECTION('',(1.,0.,0.));
#22748=DIRECTION('center_axis',(0.,1.,0.));
#22749=DIRECTION('ref_axis',(0.,0.,1.));
#22750=DIRECTION('',(0.,0.,1.));
#22751=DIRECTION('',(0.,0.,1.));
#22752=DIRECTION('',(1.,0.,0.));
#22753=DIRECTION('center_axis',(0.,0.,1.));
#22754=DIRECTION('ref_axis',(0.,-1.,0.));
#22755=DIRECTION('',(0.,-1.,0.));
#22756=DIRECTION('',(0.,-1.,0.));
#22757=DIRECTION('',(1.,0.,0.));
#22758=DIRECTION('center_axis',(0.,-1.,0.));
#22759=DIRECTION('ref_axis',(0.,0.,-1.));
#22760=DIRECTION('',(0.,0.,-1.));
#22761=DIRECTION('',(0.,0.,-1.));
#22762=DIRECTION('center_axis',(1.,0.,0.));
#22763=DIRECTION('ref_axis',(0.,0.,-1.));
#22764=DIRECTION('center_axis',(0.,0.,-1.));
#22765=DIRECTION('ref_axis',(0.,1.,0.));
#22766=DIRECTION('',(0.,1.,0.));
#22767=DIRECTION('',(1.,0.,0.));
#22768=DIRECTION('',(0.,1.,0.));
#22769=DIRECTION('',(1.,0.,0.));
#22770=DIRECTION('center_axis',(0.,1.,0.));
#22771=DIRECTION('ref_axis',(0.,0.,1.));
#22772=DIRECTION('',(0.,0.,1.));
#22773=DIRECTION('',(0.,0.,1.));
#22774=DIRECTION('',(1.,0.,0.));
#22775=DIRECTION('center_axis',(0.,0.,1.));
#22776=DIRECTION('ref_axis',(0.,-1.,0.));
#22777=DIRECTION('',(0.,-1.,0.));
#22778=DIRECTION('',(0.,-1.,0.));
#22779=DIRECTION('',(1.,0.,0.));
#22780=DIRECTION('center_axis',(0.,-1.,0.));
#22781=DIRECTION('ref_axis',(0.,0.,-1.));
#22782=DIRECTION('',(0.,0.,-1.));
#22783=DIRECTION('',(0.,0.,-1.));
#22784=DIRECTION('center_axis',(1.,0.,0.));
#22785=DIRECTION('ref_axis',(0.,0.,-1.));
#22786=DIRECTION('center_axis',(0.,0.,-1.));
#22787=DIRECTION('ref_axis',(0.,1.,0.));
#22788=DIRECTION('',(0.,1.,0.));
#22789=DIRECTION('',(1.,0.,0.));
#22790=DIRECTION('',(0.,1.,0.));
#22791=DIRECTION('',(1.,0.,0.));
#22792=DIRECTION('center_axis',(0.,1.,0.));
#22793=DIRECTION('ref_axis',(0.,0.,1.));
#22794=DIRECTION('',(0.,0.,1.));
#22795=DIRECTION('',(0.,0.,1.));
#22796=DIRECTION('',(1.,0.,0.));
#22797=DIRECTION('center_axis',(0.,0.,1.));
#22798=DIRECTION('ref_axis',(0.,-1.,0.));
#22799=DIRECTION('',(0.,-1.,0.));
#22800=DIRECTION('',(0.,-1.,0.));
#22801=DIRECTION('',(1.,0.,0.));
#22802=DIRECTION('center_axis',(0.,-1.,0.));
#22803=DIRECTION('ref_axis',(0.,0.,-1.));
#22804=DIRECTION('',(0.,0.,-1.));
#22805=DIRECTION('',(0.,0.,-1.));
#22806=DIRECTION('center_axis',(1.,0.,0.));
#22807=DIRECTION('ref_axis',(0.,0.,-1.));
#22808=DIRECTION('center_axis',(0.,0.,-1.));
#22809=DIRECTION('ref_axis',(0.,1.,0.));
#22810=DIRECTION('',(0.,1.,0.));
#22811=DIRECTION('',(1.,0.,0.));
#22812=DIRECTION('',(0.,1.,0.));
#22813=DIRECTION('',(1.,0.,0.));
#22814=DIRECTION('center_axis',(0.,1.,0.));
#22815=DIRECTION('ref_axis',(0.,0.,1.));
#22816=DIRECTION('',(0.,0.,1.));
#22817=DIRECTION('',(0.,0.,1.));
#22818=DIRECTION('',(1.,0.,0.));
#22819=DIRECTION('center_axis',(0.,0.,1.));
#22820=DIRECTION('ref_axis',(0.,-1.,0.));
#22821=DIRECTION('',(0.,-1.,0.));
#22822=DIRECTION('',(0.,-1.,0.));
#22823=DIRECTION('',(1.,0.,0.));
#22824=DIRECTION('center_axis',(0.,-1.,0.));
#22825=DIRECTION('ref_axis',(0.,0.,-1.));
#22826=DIRECTION('',(0.,0.,-1.));
#22827=DIRECTION('',(0.,0.,-1.));
#22828=DIRECTION('center_axis',(1.,0.,0.));
#22829=DIRECTION('ref_axis',(0.,0.,-1.));
#22830=DIRECTION('center_axis',(0.,0.,-1.));
#22831=DIRECTION('ref_axis',(0.,1.,0.));
#22832=DIRECTION('',(0.,1.,0.));
#22833=DIRECTION('',(1.,0.,0.));
#22834=DIRECTION('',(0.,1.,0.));
#22835=DIRECTION('',(1.,0.,0.));
#22836=DIRECTION('center_axis',(0.,1.,0.));
#22837=DIRECTION('ref_axis',(0.,0.,1.));
#22838=DIRECTION('',(0.,0.,1.));
#22839=DIRECTION('',(0.,0.,1.));
#22840=DIRECTION('',(1.,0.,0.));
#22841=DIRECTION('center_axis',(0.,0.,1.));
#22842=DIRECTION('ref_axis',(0.,-1.,0.));
#22843=DIRECTION('',(0.,-1.,0.));
#22844=DIRECTION('',(0.,-1.,0.));
#22845=DIRECTION('',(1.,0.,0.));
#22846=DIRECTION('center_axis',(0.,-1.,0.));
#22847=DIRECTION('ref_axis',(0.,0.,-1.));
#22848=DIRECTION('',(0.,0.,-1.));
#22849=DIRECTION('',(0.,0.,-1.));
#22850=DIRECTION('center_axis',(1.,0.,0.));
#22851=DIRECTION('ref_axis',(0.,0.,-1.));
#22852=DIRECTION('center_axis',(0.,0.,-1.));
#22853=DIRECTION('ref_axis',(0.,1.,0.));
#22854=DIRECTION('',(0.,1.,0.));
#22855=DIRECTION('',(1.,0.,0.));
#22856=DIRECTION('',(0.,1.,0.));
#22857=DIRECTION('',(1.,0.,0.));
#22858=DIRECTION('center_axis',(0.,1.,0.));
#22859=DIRECTION('ref_axis',(0.,0.,1.));
#22860=DIRECTION('',(0.,0.,1.));
#22861=DIRECTION('',(0.,0.,1.));
#22862=DIRECTION('',(1.,0.,0.));
#22863=DIRECTION('center_axis',(0.,0.,1.));
#22864=DIRECTION('ref_axis',(0.,-1.,0.));
#22865=DIRECTION('',(0.,-1.,0.));
#22866=DIRECTION('',(0.,-1.,0.));
#22867=DIRECTION('',(1.,0.,0.));
#22868=DIRECTION('center_axis',(0.,-1.,0.));
#22869=DIRECTION('ref_axis',(0.,0.,-1.));
#22870=DIRECTION('',(0.,0.,-1.));
#22871=DIRECTION('',(0.,0.,-1.));
#22872=DIRECTION('center_axis',(1.,0.,0.));
#22873=DIRECTION('ref_axis',(0.,0.,-1.));
#22874=DIRECTION('center_axis',(0.,0.,-1.));
#22875=DIRECTION('ref_axis',(0.,1.,0.));
#22876=DIRECTION('',(0.,1.,0.));
#22877=DIRECTION('',(1.,0.,0.));
#22878=DIRECTION('',(0.,1.,0.));
#22879=DIRECTION('',(1.,0.,0.));
#22880=DIRECTION('center_axis',(0.,1.,0.));
#22881=DIRECTION('ref_axis',(0.,0.,1.));
#22882=DIRECTION('',(0.,0.,1.));
#22883=DIRECTION('',(0.,0.,1.));
#22884=DIRECTION('',(1.,0.,0.));
#22885=DIRECTION('center_axis',(0.,0.,1.));
#22886=DIRECTION('ref_axis',(0.,-1.,0.));
#22887=DIRECTION('',(0.,-1.,0.));
#22888=DIRECTION('',(0.,-1.,0.));
#22889=DIRECTION('',(1.,0.,0.));
#22890=DIRECTION('center_axis',(0.,-1.,0.));
#22891=DIRECTION('ref_axis',(0.,0.,-1.));
#22892=DIRECTION('',(0.,0.,-1.));
#22893=DIRECTION('',(0.,0.,-1.));
#22894=DIRECTION('center_axis',(1.,0.,0.));
#22895=DIRECTION('ref_axis',(0.,0.,-1.));
#22896=DIRECTION('center_axis',(0.,0.,-1.));
#22897=DIRECTION('ref_axis',(0.,1.,0.));
#22898=DIRECTION('',(0.,1.,0.));
#22899=DIRECTION('',(1.,0.,0.));
#22900=DIRECTION('',(0.,1.,0.));
#22901=DIRECTION('',(1.,0.,0.));
#22902=DIRECTION('center_axis',(0.,1.,0.));
#22903=DIRECTION('ref_axis',(0.,0.,1.));
#22904=DIRECTION('',(0.,0.,1.));
#22905=DIRECTION('',(0.,0.,1.));
#22906=DIRECTION('',(1.,0.,0.));
#22907=DIRECTION('center_axis',(0.,0.,1.));
#22908=DIRECTION('ref_axis',(0.,-1.,0.));
#22909=DIRECTION('',(0.,-1.,0.));
#22910=DIRECTION('',(0.,-1.,0.));
#22911=DIRECTION('',(1.,0.,0.));
#22912=DIRECTION('center_axis',(0.,-1.,0.));
#22913=DIRECTION('ref_axis',(0.,0.,-1.));
#22914=DIRECTION('',(0.,0.,-1.));
#22915=DIRECTION('',(0.,0.,-1.));
#22916=DIRECTION('center_axis',(1.,0.,0.));
#22917=DIRECTION('ref_axis',(0.,0.,-1.));
#22918=DIRECTION('center_axis',(0.,0.,-1.));
#22919=DIRECTION('ref_axis',(0.,1.,0.));
#22920=DIRECTION('',(0.,1.,0.));
#22921=DIRECTION('',(1.,0.,0.));
#22922=DIRECTION('',(0.,1.,0.));
#22923=DIRECTION('',(1.,0.,0.));
#22924=DIRECTION('center_axis',(0.,1.,0.));
#22925=DIRECTION('ref_axis',(0.,0.,1.));
#22926=DIRECTION('',(0.,0.,1.));
#22927=DIRECTION('',(0.,0.,1.));
#22928=DIRECTION('',(1.,0.,0.));
#22929=DIRECTION('center_axis',(0.,0.,1.));
#22930=DIRECTION('ref_axis',(0.,-1.,0.));
#22931=DIRECTION('',(0.,-1.,0.));
#22932=DIRECTION('',(0.,-1.,0.));
#22933=DIRECTION('',(1.,0.,0.));
#22934=DIRECTION('center_axis',(0.,-1.,0.));
#22935=DIRECTION('ref_axis',(0.,0.,-1.));
#22936=DIRECTION('',(0.,0.,-1.));
#22937=DIRECTION('',(0.,0.,-1.));
#22938=DIRECTION('center_axis',(1.,0.,0.));
#22939=DIRECTION('ref_axis',(0.,0.,-1.));
#22940=DIRECTION('center_axis',(0.,0.,-1.));
#22941=DIRECTION('ref_axis',(0.,1.,0.));
#22942=DIRECTION('',(0.,1.,0.));
#22943=DIRECTION('',(1.,0.,0.));
#22944=DIRECTION('',(0.,1.,0.));
#22945=DIRECTION('',(1.,0.,0.));
#22946=DIRECTION('center_axis',(0.,1.,0.));
#22947=DIRECTION('ref_axis',(0.,0.,1.));
#22948=DIRECTION('',(0.,0.,1.));
#22949=DIRECTION('',(0.,0.,1.));
#22950=DIRECTION('',(1.,0.,0.));
#22951=DIRECTION('center_axis',(0.,0.,1.));
#22952=DIRECTION('ref_axis',(0.,-1.,0.));
#22953=DIRECTION('',(0.,-1.,0.));
#22954=DIRECTION('',(0.,-1.,0.));
#22955=DIRECTION('',(1.,0.,0.));
#22956=DIRECTION('center_axis',(0.,-1.,0.));
#22957=DIRECTION('ref_axis',(0.,0.,-1.));
#22958=DIRECTION('',(0.,0.,-1.));
#22959=DIRECTION('',(0.,0.,-1.));
#22960=DIRECTION('center_axis',(1.,0.,0.));
#22961=DIRECTION('ref_axis',(0.,0.,-1.));
#22962=DIRECTION('center_axis',(0.,0.,-1.));
#22963=DIRECTION('ref_axis',(0.,1.,0.));
#22964=DIRECTION('',(0.,1.,0.));
#22965=DIRECTION('',(1.,0.,0.));
#22966=DIRECTION('',(0.,1.,0.));
#22967=DIRECTION('',(1.,0.,0.));
#22968=DIRECTION('center_axis',(0.,1.,0.));
#22969=DIRECTION('ref_axis',(0.,0.,1.));
#22970=DIRECTION('',(0.,0.,1.));
#22971=DIRECTION('',(0.,0.,1.));
#22972=DIRECTION('',(1.,0.,0.));
#22973=DIRECTION('center_axis',(0.,0.,1.));
#22974=DIRECTION('ref_axis',(0.,-1.,0.));
#22975=DIRECTION('',(0.,-1.,0.));
#22976=DIRECTION('',(0.,-1.,0.));
#22977=DIRECTION('',(1.,0.,0.));
#22978=DIRECTION('center_axis',(0.,-1.,0.));
#22979=DIRECTION('ref_axis',(0.,0.,-1.));
#22980=DIRECTION('',(0.,0.,-1.));
#22981=DIRECTION('',(0.,0.,-1.));
#22982=DIRECTION('center_axis',(1.,0.,0.));
#22983=DIRECTION('ref_axis',(0.,0.,-1.));
#22984=DIRECTION('center_axis',(0.,0.,-1.));
#22985=DIRECTION('ref_axis',(0.,1.,0.));
#22986=DIRECTION('',(0.,1.,0.));
#22987=DIRECTION('',(1.,0.,0.));
#22988=DIRECTION('',(0.,1.,0.));
#22989=DIRECTION('',(1.,0.,0.));
#22990=DIRECTION('center_axis',(0.,1.,0.));
#22991=DIRECTION('ref_axis',(0.,0.,1.));
#22992=DIRECTION('',(0.,0.,1.));
#22993=DIRECTION('',(0.,0.,1.));
#22994=DIRECTION('',(1.,0.,0.));
#22995=DIRECTION('center_axis',(0.,0.,1.));
#22996=DIRECTION('ref_axis',(0.,-1.,0.));
#22997=DIRECTION('',(0.,-1.,0.));
#22998=DIRECTION('',(0.,-1.,0.));
#22999=DIRECTION('',(1.,0.,0.));
#23000=DIRECTION('center_axis',(0.,-1.,0.));
#23001=DIRECTION('ref_axis',(0.,0.,-1.));
#23002=DIRECTION('',(0.,0.,-1.));
#23003=DIRECTION('',(0.,0.,-1.));
#23004=DIRECTION('center_axis',(1.,0.,0.));
#23005=DIRECTION('ref_axis',(0.,0.,-1.));
#23006=DIRECTION('center_axis',(0.,0.,-1.));
#23007=DIRECTION('ref_axis',(0.,1.,0.));
#23008=DIRECTION('',(0.,1.,0.));
#23009=DIRECTION('',(1.,0.,0.));
#23010=DIRECTION('',(0.,1.,0.));
#23011=DIRECTION('',(1.,0.,0.));
#23012=DIRECTION('center_axis',(0.,1.,0.));
#23013=DIRECTION('ref_axis',(0.,0.,1.));
#23014=DIRECTION('',(0.,0.,1.));
#23015=DIRECTION('',(0.,0.,1.));
#23016=DIRECTION('',(1.,0.,0.));
#23017=DIRECTION('center_axis',(0.,0.,1.));
#23018=DIRECTION('ref_axis',(0.,-1.,0.));
#23019=DIRECTION('',(0.,-1.,0.));
#23020=DIRECTION('',(0.,-1.,0.));
#23021=DIRECTION('',(1.,0.,0.));
#23022=DIRECTION('center_axis',(0.,-1.,0.));
#23023=DIRECTION('ref_axis',(0.,0.,-1.));
#23024=DIRECTION('',(0.,0.,-1.));
#23025=DIRECTION('',(0.,0.,-1.));
#23026=DIRECTION('center_axis',(1.,0.,0.));
#23027=DIRECTION('ref_axis',(0.,0.,-1.));
#23028=DIRECTION('center_axis',(0.,0.,-1.));
#23029=DIRECTION('ref_axis',(0.,1.,0.));
#23030=DIRECTION('',(0.,1.,0.));
#23031=DIRECTION('',(1.,0.,0.));
#23032=DIRECTION('',(0.,1.,0.));
#23033=DIRECTION('',(1.,0.,0.));
#23034=DIRECTION('center_axis',(0.,1.,0.));
#23035=DIRECTION('ref_axis',(0.,0.,1.));
#23036=DIRECTION('',(0.,0.,1.));
#23037=DIRECTION('',(0.,0.,1.));
#23038=DIRECTION('',(1.,0.,0.));
#23039=DIRECTION('center_axis',(0.,0.,1.));
#23040=DIRECTION('ref_axis',(0.,-1.,0.));
#23041=DIRECTION('',(0.,-1.,0.));
#23042=DIRECTION('',(0.,-1.,0.));
#23043=DIRECTION('',(1.,0.,0.));
#23044=DIRECTION('center_axis',(0.,-1.,0.));
#23045=DIRECTION('ref_axis',(0.,0.,-1.));
#23046=DIRECTION('',(0.,0.,-1.));
#23047=DIRECTION('',(0.,0.,-1.));
#23048=DIRECTION('center_axis',(1.,0.,0.));
#23049=DIRECTION('ref_axis',(0.,0.,-1.));
#23050=DIRECTION('center_axis',(1.,0.,0.));
#23051=DIRECTION('ref_axis',(0.,0.,-1.));
#23052=DIRECTION('center_axis',(1.,0.,0.));
#23053=DIRECTION('ref_axis',(0.,0.,-1.));
#23054=DIRECTION('',(1.,0.,0.));
#23055=DIRECTION('center_axis',(-1.,0.,0.));
#23056=DIRECTION('ref_axis',(0.,0.,-1.));
#23057=DIRECTION('center_axis',(1.,0.,0.));
#23058=DIRECTION('ref_axis',(0.,0.,-1.));
#23059=DIRECTION('center_axis',(1.,0.,0.));
#23060=DIRECTION('ref_axis',(0.,0.,-1.));
#23061=DIRECTION('',(1.,0.,0.));
#23062=DIRECTION('center_axis',(-1.,0.,0.));
#23063=DIRECTION('ref_axis',(0.,0.,-1.));
#23064=DIRECTION('center_axis',(0.,1.,0.));
#23065=DIRECTION('ref_axis',(-1.,0.,0.));
#23066=DIRECTION('',(-1.,0.,0.));
#23067=DIRECTION('',(0.,0.,1.));
#23068=DIRECTION('',(-1.,0.,0.));
#23069=DIRECTION('',(0.,0.,1.));
#23070=DIRECTION('center_axis',(1.,0.,0.));
#23071=DIRECTION('ref_axis',(0.,1.,0.));
#23072=DIRECTION('',(0.,1.,0.));
#23073=DIRECTION('',(0.,1.,0.));
#23074=DIRECTION('',(0.,0.,1.));
#23075=DIRECTION('center_axis',(0.,-1.,0.));
#23076=DIRECTION('ref_axis',(1.,0.,0.));
#23077=DIRECTION('',(1.,0.,0.));
#23078=DIRECTION('',(1.,0.,0.));
#23079=DIRECTION('',(0.,0.,1.));
#23080=DIRECTION('center_axis',(-1.,0.,0.));
#23081=DIRECTION('ref_axis',(0.,-1.,0.));
#23082=DIRECTION('',(0.,-1.,0.));
#23083=DIRECTION('',(0.,-1.,0.));
#23084=DIRECTION('center_axis',(0.,0.,1.));
#23085=DIRECTION('ref_axis',(1.,0.,0.));
#23086=DIRECTION('center_axis',(0.,0.,1.));
#23087=DIRECTION('ref_axis',(1.,0.,0.));
#27612=CARTESIAN_POINT('',(0.,0.,0.));
#27613=CARTESIAN_POINT('Origin',(8.69,-0.7,21.29));
#27614=CARTESIAN_POINT('',(8.7,-0.7,21.29));
#27615=CARTESIAN_POINT('',(8.7,0.4,21.29));
#27616=CARTESIAN_POINT('',(8.7,0.05,21.29));
#27617=CARTESIAN_POINT('',(8.75,-0.7,21.29));
#27618=CARTESIAN_POINT('',(8.69,-0.7,21.29));
#27619=CARTESIAN_POINT('',(8.75,0.4,21.29));
#27620=CARTESIAN_POINT('',(8.75,-0.7,21.29));
#27621=CARTESIAN_POINT('',(8.69,0.4,21.29));
#27622=CARTESIAN_POINT('Origin',(8.69,0.4,21.29));
#27623=CARTESIAN_POINT('',(8.7,0.4,21.31));
#27624=CARTESIAN_POINT('',(8.7,0.4,11.645));
#27625=CARTESIAN_POINT('',(8.75,0.4,21.31));
#27626=CARTESIAN_POINT('',(8.75,0.4,21.29));
#27627=CARTESIAN_POINT('',(8.69,0.4,21.31));
#27628=CARTESIAN_POINT('Origin',(8.69,0.4,21.31));
#27629=CARTESIAN_POINT('',(8.7,-0.7,21.31));
#27630=CARTESIAN_POINT('',(8.7,0.6,21.31));
#27631=CARTESIAN_POINT('',(8.75,-0.7,21.31));
#27632=CARTESIAN_POINT('',(8.75,0.4,21.31));
#27633=CARTESIAN_POINT('',(8.69,-0.7,21.31));
#27634=CARTESIAN_POINT('Origin',(8.69,-0.7,21.31));
#27635=CARTESIAN_POINT('',(8.7,-0.7,11.655));
#27636=CARTESIAN_POINT('',(8.75,-0.7,21.31));
#27637=CARTESIAN_POINT('Origin',(8.75,-0.15,21.3));
#27638=CARTESIAN_POINT('Origin',(8.69,-0.7,20.79));
#27639=CARTESIAN_POINT('',(8.7,-0.7,20.79));
#27640=CARTESIAN_POINT('',(8.7,-0.1,20.79));
#27641=CARTESIAN_POINT('',(8.7,0.05,20.79));
#27642=CARTESIAN_POINT('',(8.75,-0.7,20.79));
#27643=CARTESIAN_POINT('',(8.69,-0.7,20.79));
#27644=CARTESIAN_POINT('',(8.75,-0.1,20.79));
#27645=CARTESIAN_POINT('',(8.75,-0.7,20.79));
#27646=CARTESIAN_POINT('',(8.69,-0.1,20.79));
#27647=CARTESIAN_POINT('Origin',(8.69,-0.1,20.79));
#27648=CARTESIAN_POINT('',(8.7,-0.1,20.81));
#27649=CARTESIAN_POINT('',(8.7,-0.1,11.395));
#27650=CARTESIAN_POINT('',(8.75,-0.1,20.81));
#27651=CARTESIAN_POINT('',(8.75,-0.1,20.79));
#27652=CARTESIAN_POINT('',(8.69,-0.1,20.81));
#27653=CARTESIAN_POINT('Origin',(8.69,-0.1,20.81));
#27654=CARTESIAN_POINT('',(8.7,-0.7,20.81));
#27655=CARTESIAN_POINT('',(8.7,0.35,20.81));
#27656=CARTESIAN_POINT('',(8.75,-0.7,20.81));
#27657=CARTESIAN_POINT('',(8.75,-0.1,20.81));
#27658=CARTESIAN_POINT('',(8.69,-0.7,20.81));
#27659=CARTESIAN_POINT('Origin',(8.69,-0.7,20.81));
#27660=CARTESIAN_POINT('',(8.7,-0.7,11.405));
#27661=CARTESIAN_POINT('',(8.75,-0.7,20.81));
#27662=CARTESIAN_POINT('Origin',(8.75,-0.4,20.8));
#27663=CARTESIAN_POINT('Origin',(8.69,-0.7,20.29));
#27664=CARTESIAN_POINT('',(8.7,-0.7,20.29));
#27665=CARTESIAN_POINT('',(8.7,0.4,20.29));
#27666=CARTESIAN_POINT('',(8.7,0.05,20.29));
#27667=CARTESIAN_POINT('',(8.75,-0.7,20.29));
#27668=CARTESIAN_POINT('',(8.69,-0.7,20.29));
#27669=CARTESIAN_POINT('',(8.75,0.4,20.29));
#27670=CARTESIAN_POINT('',(8.75,-0.7,20.29));
#27671=CARTESIAN_POINT('',(8.69,0.4,20.29));
#27672=CARTESIAN_POINT('Origin',(8.69,0.4,20.29));
#27673=CARTESIAN_POINT('',(8.7,0.4,20.31));
#27674=CARTESIAN_POINT('',(8.7,0.4,11.145));
#27675=CARTESIAN_POINT('',(8.75,0.4,20.31));
#27676=CARTESIAN_POINT('',(8.75,0.4,20.29));
#27677=CARTESIAN_POINT('',(8.69,0.4,20.31));
#27678=CARTESIAN_POINT('Origin',(8.69,0.4,20.31));
#27679=CARTESIAN_POINT('',(8.7,-0.7,20.31));
#27680=CARTESIAN_POINT('',(8.7,0.6,20.31));
#27681=CARTESIAN_POINT('',(8.75,-0.7,20.31));
#27682=CARTESIAN_POINT('',(8.75,0.4,20.31));
#27683=CARTESIAN_POINT('',(8.69,-0.7,20.31));
#27684=CARTESIAN_POINT('Origin',(8.69,-0.7,20.31));
#27685=CARTESIAN_POINT('',(8.7,-0.7,11.155));
#27686=CARTESIAN_POINT('',(8.75,-0.7,20.31));
#27687=CARTESIAN_POINT('Origin',(8.75,-0.15,20.3));
#27688=CARTESIAN_POINT('Origin',(8.69,-0.7,19.79));
#27689=CARTESIAN_POINT('',(8.7,-0.7,19.79));
#27690=CARTESIAN_POINT('',(8.7,-0.1,19.79));
#27691=CARTESIAN_POINT('',(8.7,0.05,19.79));
#27692=CARTESIAN_POINT('',(8.75,-0.7,19.79));
#27693=CARTESIAN_POINT('',(8.69,-0.7,19.79));
#27694=CARTESIAN_POINT('',(8.75,-0.1,19.79));
#27695=CARTESIAN_POINT('',(8.75,-0.7,19.79));
#27696=CARTESIAN_POINT('',(8.69,-0.1,19.79));
#27697=CARTESIAN_POINT('Origin',(8.69,-0.1,19.79));
#27698=CARTESIAN_POINT('',(8.7,-0.1,19.81));
#27699=CARTESIAN_POINT('',(8.7,-0.1,10.895));
#27700=CARTESIAN_POINT('',(8.75,-0.1,19.81));
#27701=CARTESIAN_POINT('',(8.75,-0.1,19.79));
#27702=CARTESIAN_POINT('',(8.69,-0.1,19.81));
#27703=CARTESIAN_POINT('Origin',(8.69,-0.1,19.81));
#27704=CARTESIAN_POINT('',(8.7,-0.7,19.81));
#27705=CARTESIAN_POINT('',(8.7,0.35,19.81));
#27706=CARTESIAN_POINT('',(8.75,-0.7,19.81));
#27707=CARTESIAN_POINT('',(8.75,-0.1,19.81));
#27708=CARTESIAN_POINT('',(8.69,-0.7,19.81));
#27709=CARTESIAN_POINT('Origin',(8.69,-0.7,19.81));
#27710=CARTESIAN_POINT('',(8.7,-0.7,10.905));
#27711=CARTESIAN_POINT('',(8.75,-0.7,19.81));
#27712=CARTESIAN_POINT('Origin',(8.75,-0.4,19.8));
#27713=CARTESIAN_POINT('Origin',(8.69,-0.7,19.29));
#27714=CARTESIAN_POINT('',(8.7,-0.7,19.29));
#27715=CARTESIAN_POINT('',(8.7,0.4,19.29));
#27716=CARTESIAN_POINT('',(8.7,0.05,19.29));
#27717=CARTESIAN_POINT('',(8.75,-0.7,19.29));
#27718=CARTESIAN_POINT('',(8.69,-0.7,19.29));
#27719=CARTESIAN_POINT('',(8.75,0.4,19.29));
#27720=CARTESIAN_POINT('',(8.75,-0.7,19.29));
#27721=CARTESIAN_POINT('',(8.69,0.4,19.29));
#27722=CARTESIAN_POINT('Origin',(8.69,0.4,19.29));
#27723=CARTESIAN_POINT('',(8.7,0.4,19.31));
#27724=CARTESIAN_POINT('',(8.7,0.4,10.645));
#27725=CARTESIAN_POINT('',(8.75,0.4,19.31));
#27726=CARTESIAN_POINT('',(8.75,0.4,19.29));
#27727=CARTESIAN_POINT('',(8.69,0.4,19.31));
#27728=CARTESIAN_POINT('Origin',(8.69,0.4,19.31));
#27729=CARTESIAN_POINT('',(8.7,-0.7,19.31));
#27730=CARTESIAN_POINT('',(8.7,0.6,19.31));
#27731=CARTESIAN_POINT('',(8.75,-0.7,19.31));
#27732=CARTESIAN_POINT('',(8.75,0.4,19.31));
#27733=CARTESIAN_POINT('',(8.69,-0.7,19.31));
#27734=CARTESIAN_POINT('Origin',(8.69,-0.7,19.31));
#27735=CARTESIAN_POINT('',(8.7,-0.7,10.655));
#27736=CARTESIAN_POINT('',(8.75,-0.7,19.31));
#27737=CARTESIAN_POINT('Origin',(8.75,-0.15,19.3));
#27738=CARTESIAN_POINT('Origin',(8.69,-0.7,18.79));
#27739=CARTESIAN_POINT('',(8.7,-0.7,18.79));
#27740=CARTESIAN_POINT('',(8.7,-0.1,18.79));
#27741=CARTESIAN_POINT('',(8.7,0.05,18.79));
#27742=CARTESIAN_POINT('',(8.75,-0.7,18.79));
#27743=CARTESIAN_POINT('',(8.69,-0.7,18.79));
#27744=CARTESIAN_POINT('',(8.75,-0.1,18.79));
#27745=CARTESIAN_POINT('',(8.75,-0.7,18.79));
#27746=CARTESIAN_POINT('',(8.69,-0.1,18.79));
#27747=CARTESIAN_POINT('Origin',(8.69,-0.1,18.79));
#27748=CARTESIAN_POINT('',(8.7,-0.1,18.81));
#27749=CARTESIAN_POINT('',(8.7,-0.1,10.395));
#27750=CARTESIAN_POINT('',(8.75,-0.1,18.81));
#27751=CARTESIAN_POINT('',(8.75,-0.1,18.79));
#27752=CARTESIAN_POINT('',(8.69,-0.1,18.81));
#27753=CARTESIAN_POINT('Origin',(8.69,-0.1,18.81));
#27754=CARTESIAN_POINT('',(8.7,-0.7,18.81));
#27755=CARTESIAN_POINT('',(8.7,0.35,18.81));
#27756=CARTESIAN_POINT('',(8.75,-0.7,18.81));
#27757=CARTESIAN_POINT('',(8.75,-0.1,18.81));
#27758=CARTESIAN_POINT('',(8.69,-0.7,18.81));
#27759=CARTESIAN_POINT('Origin',(8.69,-0.7,18.81));
#27760=CARTESIAN_POINT('',(8.7,-0.7,10.405));
#27761=CARTESIAN_POINT('',(8.75,-0.7,18.81));
#27762=CARTESIAN_POINT('Origin',(8.75,-0.4,18.8));
#27763=CARTESIAN_POINT('Origin',(8.69,-0.7,18.29));
#27764=CARTESIAN_POINT('',(8.7,-0.7,18.29));
#27765=CARTESIAN_POINT('',(8.7,0.4,18.29));
#27766=CARTESIAN_POINT('',(8.7,0.05,18.29));
#27767=CARTESIAN_POINT('',(8.75,-0.7,18.29));
#27768=CARTESIAN_POINT('',(8.69,-0.7,18.29));
#27769=CARTESIAN_POINT('',(8.75,0.4,18.29));
#27770=CARTESIAN_POINT('',(8.75,-0.7,18.29));
#27771=CARTESIAN_POINT('',(8.69,0.4,18.29));
#27772=CARTESIAN_POINT('Origin',(8.69,0.4,18.29));
#27773=CARTESIAN_POINT('',(8.7,0.4,18.31));
#27774=CARTESIAN_POINT('',(8.7,0.4,10.145));
#27775=CARTESIAN_POINT('',(8.75,0.4,18.31));
#27776=CARTESIAN_POINT('',(8.75,0.4,18.29));
#27777=CARTESIAN_POINT('',(8.69,0.4,18.31));
#27778=CARTESIAN_POINT('Origin',(8.69,0.4,18.31));
#27779=CARTESIAN_POINT('',(8.7,-0.7,18.31));
#27780=CARTESIAN_POINT('',(8.7,0.6,18.31));
#27781=CARTESIAN_POINT('',(8.75,-0.7,18.31));
#27782=CARTESIAN_POINT('',(8.75,0.4,18.31));
#27783=CARTESIAN_POINT('',(8.69,-0.7,18.31));
#27784=CARTESIAN_POINT('Origin',(8.69,-0.7,18.31));
#27785=CARTESIAN_POINT('',(8.7,-0.7,10.155));
#27786=CARTESIAN_POINT('',(8.75,-0.7,18.31));
#27787=CARTESIAN_POINT('Origin',(8.75,-0.15,18.3));
#27788=CARTESIAN_POINT('Origin',(8.69,-0.7,17.79));
#27789=CARTESIAN_POINT('',(8.7,-0.7,17.79));
#27790=CARTESIAN_POINT('',(8.7,-0.1,17.79));
#27791=CARTESIAN_POINT('',(8.7,0.05,17.79));
#27792=CARTESIAN_POINT('',(8.75,-0.7,17.79));
#27793=CARTESIAN_POINT('',(8.69,-0.7,17.79));
#27794=CARTESIAN_POINT('',(8.75,-0.1,17.79));
#27795=CARTESIAN_POINT('',(8.75,-0.7,17.79));
#27796=CARTESIAN_POINT('',(8.69,-0.1,17.79));
#27797=CARTESIAN_POINT('Origin',(8.69,-0.1,17.79));
#27798=CARTESIAN_POINT('',(8.7,-0.1,17.81));
#27799=CARTESIAN_POINT('',(8.7,-0.1,9.895));
#27800=CARTESIAN_POINT('',(8.75,-0.1,17.81));
#27801=CARTESIAN_POINT('',(8.75,-0.1,17.79));
#27802=CARTESIAN_POINT('',(8.69,-0.1,17.81));
#27803=CARTESIAN_POINT('Origin',(8.69,-0.1,17.81));
#27804=CARTESIAN_POINT('',(8.7,-0.7,17.81));
#27805=CARTESIAN_POINT('',(8.7,0.35,17.81));
#27806=CARTESIAN_POINT('',(8.75,-0.7,17.81));
#27807=CARTESIAN_POINT('',(8.75,-0.1,17.81));
#27808=CARTESIAN_POINT('',(8.69,-0.7,17.81));
#27809=CARTESIAN_POINT('Origin',(8.69,-0.7,17.81));
#27810=CARTESIAN_POINT('',(8.7,-0.7,9.905));
#27811=CARTESIAN_POINT('',(8.75,-0.7,17.81));
#27812=CARTESIAN_POINT('Origin',(8.75,-0.4,17.8));
#27813=CARTESIAN_POINT('Origin',(8.69,-0.7,17.29));
#27814=CARTESIAN_POINT('',(8.7,-0.7,17.29));
#27815=CARTESIAN_POINT('',(8.7,0.4,17.29));
#27816=CARTESIAN_POINT('',(8.7,0.05,17.29));
#27817=CARTESIAN_POINT('',(8.75,-0.7,17.29));
#27818=CARTESIAN_POINT('',(8.69,-0.7,17.29));
#27819=CARTESIAN_POINT('',(8.75,0.4,17.29));
#27820=CARTESIAN_POINT('',(8.75,-0.7,17.29));
#27821=CARTESIAN_POINT('',(8.69,0.4,17.29));
#27822=CARTESIAN_POINT('Origin',(8.69,0.4,17.29));
#27823=CARTESIAN_POINT('',(8.7,0.4,17.31));
#27824=CARTESIAN_POINT('',(8.7,0.4,9.645));
#27825=CARTESIAN_POINT('',(8.75,0.4,17.31));
#27826=CARTESIAN_POINT('',(8.75,0.4,17.29));
#27827=CARTESIAN_POINT('',(8.69,0.4,17.31));
#27828=CARTESIAN_POINT('Origin',(8.69,0.4,17.31));
#27829=CARTESIAN_POINT('',(8.7,-0.7,17.31));
#27830=CARTESIAN_POINT('',(8.7,0.6,17.31));
#27831=CARTESIAN_POINT('',(8.75,-0.7,17.31));
#27832=CARTESIAN_POINT('',(8.75,0.4,17.31));
#27833=CARTESIAN_POINT('',(8.69,-0.7,17.31));
#27834=CARTESIAN_POINT('Origin',(8.69,-0.7,17.31));
#27835=CARTESIAN_POINT('',(8.7,-0.7,9.655));
#27836=CARTESIAN_POINT('',(8.75,-0.7,17.31));
#27837=CARTESIAN_POINT('Origin',(8.75,-0.15,17.3));
#27838=CARTESIAN_POINT('Origin',(8.69,-0.7,16.79));
#27839=CARTESIAN_POINT('',(8.7,-0.7,16.79));
#27840=CARTESIAN_POINT('',(8.7,-0.1,16.79));
#27841=CARTESIAN_POINT('',(8.7,0.05,16.79));
#27842=CARTESIAN_POINT('',(8.75,-0.7,16.79));
#27843=CARTESIAN_POINT('',(8.69,-0.7,16.79));
#27844=CARTESIAN_POINT('',(8.75,-0.1,16.79));
#27845=CARTESIAN_POINT('',(8.75,-0.7,16.79));
#27846=CARTESIAN_POINT('',(8.69,-0.1,16.79));
#27847=CARTESIAN_POINT('Origin',(8.69,-0.1,16.79));
#27848=CARTESIAN_POINT('',(8.7,-0.1,16.81));
#27849=CARTESIAN_POINT('',(8.7,-0.1,9.395));
#27850=CARTESIAN_POINT('',(8.75,-0.1,16.81));
#27851=CARTESIAN_POINT('',(8.75,-0.1,16.79));
#27852=CARTESIAN_POINT('',(8.69,-0.1,16.81));
#27853=CARTESIAN_POINT('Origin',(8.69,-0.1,16.81));
#27854=CARTESIAN_POINT('',(8.7,-0.7,16.81));
#27855=CARTESIAN_POINT('',(8.7,0.35,16.81));
#27856=CARTESIAN_POINT('',(8.75,-0.7,16.81));
#27857=CARTESIAN_POINT('',(8.75,-0.1,16.81));
#27858=CARTESIAN_POINT('',(8.69,-0.7,16.81));
#27859=CARTESIAN_POINT('Origin',(8.69,-0.7,16.81));
#27860=CARTESIAN_POINT('',(8.7,-0.7,9.405));
#27861=CARTESIAN_POINT('',(8.75,-0.7,16.81));
#27862=CARTESIAN_POINT('Origin',(8.75,-0.4,16.8));
#27863=CARTESIAN_POINT('Origin',(8.69,-0.7,16.29));
#27864=CARTESIAN_POINT('',(8.7,-0.7,16.29));
#27865=CARTESIAN_POINT('',(8.7,0.4,16.29));
#27866=CARTESIAN_POINT('',(8.7,0.05,16.29));
#27867=CARTESIAN_POINT('',(8.75,-0.7,16.29));
#27868=CARTESIAN_POINT('',(8.69,-0.7,16.29));
#27869=CARTESIAN_POINT('',(8.75,0.4,16.29));
#27870=CARTESIAN_POINT('',(8.75,-0.7,16.29));
#27871=CARTESIAN_POINT('',(8.69,0.4,16.29));
#27872=CARTESIAN_POINT('Origin',(8.69,0.4,16.29));
#27873=CARTESIAN_POINT('',(8.7,0.4,16.31));
#27874=CARTESIAN_POINT('',(8.7,0.4,9.145));
#27875=CARTESIAN_POINT('',(8.75,0.4,16.31));
#27876=CARTESIAN_POINT('',(8.75,0.4,16.29));
#27877=CARTESIAN_POINT('',(8.69,0.4,16.31));
#27878=CARTESIAN_POINT('Origin',(8.69,0.4,16.31));
#27879=CARTESIAN_POINT('',(8.7,-0.7,16.31));
#27880=CARTESIAN_POINT('',(8.7,0.6,16.31));
#27881=CARTESIAN_POINT('',(8.75,-0.7,16.31));
#27882=CARTESIAN_POINT('',(8.75,0.4,16.31));
#27883=CARTESIAN_POINT('',(8.69,-0.7,16.31));
#27884=CARTESIAN_POINT('Origin',(8.69,-0.7,16.31));
#27885=CARTESIAN_POINT('',(8.7,-0.7,9.155));
#27886=CARTESIAN_POINT('',(8.75,-0.7,16.31));
#27887=CARTESIAN_POINT('Origin',(8.75,-0.15,16.3));
#27888=CARTESIAN_POINT('Origin',(8.69,-0.7,15.79));
#27889=CARTESIAN_POINT('',(8.7,-0.7,15.79));
#27890=CARTESIAN_POINT('',(8.7,-0.1,15.79));
#27891=CARTESIAN_POINT('',(8.7,0.05,15.79));
#27892=CARTESIAN_POINT('',(8.75,-0.7,15.79));
#27893=CARTESIAN_POINT('',(8.69,-0.7,15.79));
#27894=CARTESIAN_POINT('',(8.75,-0.1,15.79));
#27895=CARTESIAN_POINT('',(8.75,-0.7,15.79));
#27896=CARTESIAN_POINT('',(8.69,-0.1,15.79));
#27897=CARTESIAN_POINT('Origin',(8.69,-0.1,15.79));
#27898=CARTESIAN_POINT('',(8.7,-0.1,15.81));
#27899=CARTESIAN_POINT('',(8.7,-0.1,8.895));
#27900=CARTESIAN_POINT('',(8.75,-0.1,15.81));
#27901=CARTESIAN_POINT('',(8.75,-0.1,15.79));
#27902=CARTESIAN_POINT('',(8.69,-0.1,15.81));
#27903=CARTESIAN_POINT('Origin',(8.69,-0.1,15.81));
#27904=CARTESIAN_POINT('',(8.7,-0.7,15.81));
#27905=CARTESIAN_POINT('',(8.7,0.35,15.81));
#27906=CARTESIAN_POINT('',(8.75,-0.7,15.81));
#27907=CARTESIAN_POINT('',(8.75,-0.1,15.81));
#27908=CARTESIAN_POINT('',(8.69,-0.7,15.81));
#27909=CARTESIAN_POINT('Origin',(8.69,-0.7,15.81));
#27910=CARTESIAN_POINT('',(8.7,-0.7,8.905));
#27911=CARTESIAN_POINT('',(8.75,-0.7,15.81));
#27912=CARTESIAN_POINT('Origin',(8.75,-0.4,15.8));
#27913=CARTESIAN_POINT('Origin',(8.69,-0.7,15.29));
#27914=CARTESIAN_POINT('',(8.7,-0.7,15.29));
#27915=CARTESIAN_POINT('',(8.7,0.4,15.29));
#27916=CARTESIAN_POINT('',(8.7,0.05,15.29));
#27917=CARTESIAN_POINT('',(8.75,-0.7,15.29));
#27918=CARTESIAN_POINT('',(8.69,-0.7,15.29));
#27919=CARTESIAN_POINT('',(8.75,0.4,15.29));
#27920=CARTESIAN_POINT('',(8.75,-0.7,15.29));
#27921=CARTESIAN_POINT('',(8.69,0.4,15.29));
#27922=CARTESIAN_POINT('Origin',(8.69,0.4,15.29));
#27923=CARTESIAN_POINT('',(8.7,0.4,15.31));
#27924=CARTESIAN_POINT('',(8.7,0.4,8.645));
#27925=CARTESIAN_POINT('',(8.75,0.4,15.31));
#27926=CARTESIAN_POINT('',(8.75,0.4,15.29));
#27927=CARTESIAN_POINT('',(8.69,0.4,15.31));
#27928=CARTESIAN_POINT('Origin',(8.69,0.4,15.31));
#27929=CARTESIAN_POINT('',(8.7,-0.7,15.31));
#27930=CARTESIAN_POINT('',(8.7,0.6,15.31));
#27931=CARTESIAN_POINT('',(8.75,-0.7,15.31));
#27932=CARTESIAN_POINT('',(8.75,0.4,15.31));
#27933=CARTESIAN_POINT('',(8.69,-0.7,15.31));
#27934=CARTESIAN_POINT('Origin',(8.69,-0.7,15.31));
#27935=CARTESIAN_POINT('',(8.7,-0.7,8.655));
#27936=CARTESIAN_POINT('',(8.75,-0.7,15.31));
#27937=CARTESIAN_POINT('Origin',(8.75,-0.15,15.3));
#27938=CARTESIAN_POINT('Origin',(8.69,-0.7,14.79));
#27939=CARTESIAN_POINT('',(8.7,-0.7,14.79));
#27940=CARTESIAN_POINT('',(8.7,-0.1,14.79));
#27941=CARTESIAN_POINT('',(8.7,0.05,14.79));
#27942=CARTESIAN_POINT('',(8.75,-0.7,14.79));
#27943=CARTESIAN_POINT('',(8.69,-0.7,14.79));
#27944=CARTESIAN_POINT('',(8.75,-0.1,14.79));
#27945=CARTESIAN_POINT('',(8.75,-0.7,14.79));
#27946=CARTESIAN_POINT('',(8.69,-0.1,14.79));
#27947=CARTESIAN_POINT('Origin',(8.69,-0.1,14.79));
#27948=CARTESIAN_POINT('',(8.7,-0.1,14.81));
#27949=CARTESIAN_POINT('',(8.7,-0.1,8.395));
#27950=CARTESIAN_POINT('',(8.75,-0.1,14.81));
#27951=CARTESIAN_POINT('',(8.75,-0.1,14.79));
#27952=CARTESIAN_POINT('',(8.69,-0.1,14.81));
#27953=CARTESIAN_POINT('Origin',(8.69,-0.1,14.81));
#27954=CARTESIAN_POINT('',(8.7,-0.7,14.81));
#27955=CARTESIAN_POINT('',(8.7,0.35,14.81));
#27956=CARTESIAN_POINT('',(8.75,-0.7,14.81));
#27957=CARTESIAN_POINT('',(8.75,-0.1,14.81));
#27958=CARTESIAN_POINT('',(8.69,-0.7,14.81));
#27959=CARTESIAN_POINT('Origin',(8.69,-0.7,14.81));
#27960=CARTESIAN_POINT('',(8.7,-0.7,8.405));
#27961=CARTESIAN_POINT('',(8.75,-0.7,14.81));
#27962=CARTESIAN_POINT('Origin',(8.75,-0.4,14.8));
#27963=CARTESIAN_POINT('Origin',(8.69,-0.7,14.29));
#27964=CARTESIAN_POINT('',(8.7,-0.7,14.29));
#27965=CARTESIAN_POINT('',(8.7,0.4,14.29));
#27966=CARTESIAN_POINT('',(8.7,0.05,14.29));
#27967=CARTESIAN_POINT('',(8.75,-0.7,14.29));
#27968=CARTESIAN_POINT('',(8.69,-0.7,14.29));
#27969=CARTESIAN_POINT('',(8.75,0.4,14.29));
#27970=CARTESIAN_POINT('',(8.75,-0.7,14.29));
#27971=CARTESIAN_POINT('',(8.69,0.4,14.29));
#27972=CARTESIAN_POINT('Origin',(8.69,0.4,14.29));
#27973=CARTESIAN_POINT('',(8.7,0.4,14.31));
#27974=CARTESIAN_POINT('',(8.7,0.4,8.145));
#27975=CARTESIAN_POINT('',(8.75,0.4,14.31));
#27976=CARTESIAN_POINT('',(8.75,0.4,14.29));
#27977=CARTESIAN_POINT('',(8.69,0.4,14.31));
#27978=CARTESIAN_POINT('Origin',(8.69,0.4,14.31));
#27979=CARTESIAN_POINT('',(8.7,-0.7,14.31));
#27980=CARTESIAN_POINT('',(8.7,0.6,14.31));
#27981=CARTESIAN_POINT('',(8.75,-0.7,14.31));
#27982=CARTESIAN_POINT('',(8.75,0.4,14.31));
#27983=CARTESIAN_POINT('',(8.69,-0.7,14.31));
#27984=CARTESIAN_POINT('Origin',(8.69,-0.7,14.31));
#27985=CARTESIAN_POINT('',(8.7,-0.7,8.155));
#27986=CARTESIAN_POINT('',(8.75,-0.7,14.31));
#27987=CARTESIAN_POINT('Origin',(8.75,-0.15,14.3));
#27988=CARTESIAN_POINT('Origin',(8.69,-0.7,13.79));
#27989=CARTESIAN_POINT('',(8.7,-0.7,13.79));
#27990=CARTESIAN_POINT('',(8.7,-0.1,13.79));
#27991=CARTESIAN_POINT('',(8.7,0.05,13.79));
#27992=CARTESIAN_POINT('',(8.75,-0.7,13.79));
#27993=CARTESIAN_POINT('',(8.69,-0.7,13.79));
#27994=CARTESIAN_POINT('',(8.75,-0.1,13.79));
#27995=CARTESIAN_POINT('',(8.75,-0.7,13.79));
#27996=CARTESIAN_POINT('',(8.69,-0.1,13.79));
#27997=CARTESIAN_POINT('Origin',(8.69,-0.1,13.79));
#27998=CARTESIAN_POINT('',(8.7,-0.1,13.81));
#27999=CARTESIAN_POINT('',(8.7,-0.1,7.895));
#28000=CARTESIAN_POINT('',(8.75,-0.1,13.81));
#28001=CARTESIAN_POINT('',(8.75,-0.1,13.79));
#28002=CARTESIAN_POINT('',(8.69,-0.1,13.81));
#28003=CARTESIAN_POINT('Origin',(8.69,-0.1,13.81));
#28004=CARTESIAN_POINT('',(8.7,-0.7,13.81));
#28005=CARTESIAN_POINT('',(8.7,0.35,13.81));
#28006=CARTESIAN_POINT('',(8.75,-0.7,13.81));
#28007=CARTESIAN_POINT('',(8.75,-0.1,13.81));
#28008=CARTESIAN_POINT('',(8.69,-0.7,13.81));
#28009=CARTESIAN_POINT('Origin',(8.69,-0.7,13.81));
#28010=CARTESIAN_POINT('',(8.7,-0.7,7.905));
#28011=CARTESIAN_POINT('',(8.75,-0.7,13.81));
#28012=CARTESIAN_POINT('Origin',(8.75,-0.4,13.8));
#28013=CARTESIAN_POINT('Origin',(8.69,-0.7,13.29));
#28014=CARTESIAN_POINT('',(8.7,-0.7,13.29));
#28015=CARTESIAN_POINT('',(8.7,0.4,13.29));
#28016=CARTESIAN_POINT('',(8.7,0.05,13.29));
#28017=CARTESIAN_POINT('',(8.75,-0.7,13.29));
#28018=CARTESIAN_POINT('',(8.69,-0.7,13.29));
#28019=CARTESIAN_POINT('',(8.75,0.4,13.29));
#28020=CARTESIAN_POINT('',(8.75,-0.7,13.29));
#28021=CARTESIAN_POINT('',(8.69,0.4,13.29));
#28022=CARTESIAN_POINT('Origin',(8.69,0.4,13.29));
#28023=CARTESIAN_POINT('',(8.7,0.4,13.31));
#28024=CARTESIAN_POINT('',(8.7,0.4,7.645));
#28025=CARTESIAN_POINT('',(8.75,0.4,13.31));
#28026=CARTESIAN_POINT('',(8.75,0.4,13.29));
#28027=CARTESIAN_POINT('',(8.69,0.4,13.31));
#28028=CARTESIAN_POINT('Origin',(8.69,0.4,13.31));
#28029=CARTESIAN_POINT('',(8.7,-0.7,13.31));
#28030=CARTESIAN_POINT('',(8.7,0.6,13.31));
#28031=CARTESIAN_POINT('',(8.75,-0.7,13.31));
#28032=CARTESIAN_POINT('',(8.75,0.4,13.31));
#28033=CARTESIAN_POINT('',(8.69,-0.7,13.31));
#28034=CARTESIAN_POINT('Origin',(8.69,-0.7,13.31));
#28035=CARTESIAN_POINT('',(8.7,-0.7,7.655));
#28036=CARTESIAN_POINT('',(8.75,-0.7,13.31));
#28037=CARTESIAN_POINT('Origin',(8.75,-0.15,13.3));
#28038=CARTESIAN_POINT('Origin',(8.69,-0.7,12.79));
#28039=CARTESIAN_POINT('',(8.7,-0.7,12.79));
#28040=CARTESIAN_POINT('',(8.7,-0.1,12.79));
#28041=CARTESIAN_POINT('',(8.7,0.05,12.79));
#28042=CARTESIAN_POINT('',(8.75,-0.7,12.79));
#28043=CARTESIAN_POINT('',(8.69,-0.7,12.79));
#28044=CARTESIAN_POINT('',(8.75,-0.1,12.79));
#28045=CARTESIAN_POINT('',(8.75,-0.7,12.79));
#28046=CARTESIAN_POINT('',(8.69,-0.1,12.79));
#28047=CARTESIAN_POINT('Origin',(8.69,-0.1,12.79));
#28048=CARTESIAN_POINT('',(8.7,-0.1,12.81));
#28049=CARTESIAN_POINT('',(8.7,-0.1,7.395));
#28050=CARTESIAN_POINT('',(8.75,-0.1,12.81));
#28051=CARTESIAN_POINT('',(8.75,-0.1,12.79));
#28052=CARTESIAN_POINT('',(8.69,-0.1,12.81));
#28053=CARTESIAN_POINT('Origin',(8.69,-0.1,12.81));
#28054=CARTESIAN_POINT('',(8.7,-0.7,12.81));
#28055=CARTESIAN_POINT('',(8.7,0.35,12.81));
#28056=CARTESIAN_POINT('',(8.75,-0.7,12.81));
#28057=CARTESIAN_POINT('',(8.75,-0.1,12.81));
#28058=CARTESIAN_POINT('',(8.69,-0.7,12.81));
#28059=CARTESIAN_POINT('Origin',(8.69,-0.7,12.81));
#28060=CARTESIAN_POINT('',(8.7,-0.7,7.405));
#28061=CARTESIAN_POINT('',(8.75,-0.7,12.81));
#28062=CARTESIAN_POINT('Origin',(8.75,-0.4,12.8));
#28063=CARTESIAN_POINT('Origin',(8.69,-0.7,12.29));
#28064=CARTESIAN_POINT('',(8.7,-0.7,12.29));
#28065=CARTESIAN_POINT('',(8.7,0.4,12.29));
#28066=CARTESIAN_POINT('',(8.7,0.05,12.29));
#28067=CARTESIAN_POINT('',(8.75,-0.7,12.29));
#28068=CARTESIAN_POINT('',(8.69,-0.7,12.29));
#28069=CARTESIAN_POINT('',(8.75,0.4,12.29));
#28070=CARTESIAN_POINT('',(8.75,-0.7,12.29));
#28071=CARTESIAN_POINT('',(8.69,0.4,12.29));
#28072=CARTESIAN_POINT('Origin',(8.69,0.4,12.29));
#28073=CARTESIAN_POINT('',(8.7,0.4,12.31));
#28074=CARTESIAN_POINT('',(8.7,0.4,7.145));
#28075=CARTESIAN_POINT('',(8.75,0.4,12.31));
#28076=CARTESIAN_POINT('',(8.75,0.4,12.29));
#28077=CARTESIAN_POINT('',(8.69,0.4,12.31));
#28078=CARTESIAN_POINT('Origin',(8.69,0.4,12.31));
#28079=CARTESIAN_POINT('',(8.7,-0.7,12.31));
#28080=CARTESIAN_POINT('',(8.7,0.6,12.31));
#28081=CARTESIAN_POINT('',(8.75,-0.7,12.31));
#28082=CARTESIAN_POINT('',(8.75,0.4,12.31));
#28083=CARTESIAN_POINT('',(8.69,-0.7,12.31));
#28084=CARTESIAN_POINT('Origin',(8.69,-0.7,12.31));
#28085=CARTESIAN_POINT('',(8.7,-0.7,7.155));
#28086=CARTESIAN_POINT('',(8.75,-0.7,12.31));
#28087=CARTESIAN_POINT('Origin',(8.75,-0.15,12.3));
#28088=CARTESIAN_POINT('Origin',(8.69,-0.7,11.79));
#28089=CARTESIAN_POINT('',(8.7,-0.7,11.79));
#28090=CARTESIAN_POINT('',(8.7,-0.1,11.79));
#28091=CARTESIAN_POINT('',(8.7,0.05,11.79));
#28092=CARTESIAN_POINT('',(8.75,-0.7,11.79));
#28093=CARTESIAN_POINT('',(8.69,-0.7,11.79));
#28094=CARTESIAN_POINT('',(8.75,-0.1,11.79));
#28095=CARTESIAN_POINT('',(8.75,-0.7,11.79));
#28096=CARTESIAN_POINT('',(8.69,-0.1,11.79));
#28097=CARTESIAN_POINT('Origin',(8.69,-0.1,11.79));
#28098=CARTESIAN_POINT('',(8.7,-0.1,11.81));
#28099=CARTESIAN_POINT('',(8.7,-0.1,6.895));
#28100=CARTESIAN_POINT('',(8.75,-0.1,11.81));
#28101=CARTESIAN_POINT('',(8.75,-0.1,11.79));
#28102=CARTESIAN_POINT('',(8.69,-0.1,11.81));
#28103=CARTESIAN_POINT('Origin',(8.69,-0.1,11.81));
#28104=CARTESIAN_POINT('',(8.7,-0.7,11.81));
#28105=CARTESIAN_POINT('',(8.7,0.35,11.81));
#28106=CARTESIAN_POINT('',(8.75,-0.7,11.81));
#28107=CARTESIAN_POINT('',(8.75,-0.1,11.81));
#28108=CARTESIAN_POINT('',(8.69,-0.7,11.81));
#28109=CARTESIAN_POINT('Origin',(8.69,-0.7,11.81));
#28110=CARTESIAN_POINT('',(8.7,-0.7,6.905));
#28111=CARTESIAN_POINT('',(8.75,-0.7,11.81));
#28112=CARTESIAN_POINT('Origin',(8.75,-0.4,11.8));
#28113=CARTESIAN_POINT('Origin',(8.69,-0.7,11.29));
#28114=CARTESIAN_POINT('',(8.7,-0.7,11.29));
#28115=CARTESIAN_POINT('',(8.7,0.4,11.29));
#28116=CARTESIAN_POINT('',(8.7,0.05,11.29));
#28117=CARTESIAN_POINT('',(8.75,-0.7,11.29));
#28118=CARTESIAN_POINT('',(8.69,-0.7,11.29));
#28119=CARTESIAN_POINT('',(8.75,0.4,11.29));
#28120=CARTESIAN_POINT('',(8.75,-0.7,11.29));
#28121=CARTESIAN_POINT('',(8.69,0.4,11.29));
#28122=CARTESIAN_POINT('Origin',(8.69,0.4,11.29));
#28123=CARTESIAN_POINT('',(8.7,0.4,11.31));
#28124=CARTESIAN_POINT('',(8.7,0.4,6.645));
#28125=CARTESIAN_POINT('',(8.75,0.4,11.31));
#28126=CARTESIAN_POINT('',(8.75,0.4,11.29));
#28127=CARTESIAN_POINT('',(8.69,0.4,11.31));
#28128=CARTESIAN_POINT('Origin',(8.69,0.4,11.31));
#28129=CARTESIAN_POINT('',(8.7,-0.7,11.31));
#28130=CARTESIAN_POINT('',(8.7,0.6,11.31));
#28131=CARTESIAN_POINT('',(8.75,-0.7,11.31));
#28132=CARTESIAN_POINT('',(8.75,0.4,11.31));
#28133=CARTESIAN_POINT('',(8.69,-0.7,11.31));
#28134=CARTESIAN_POINT('Origin',(8.69,-0.7,11.31));
#28135=CARTESIAN_POINT('',(8.7,-0.7,6.655));
#28136=CARTESIAN_POINT('',(8.75,-0.7,11.31));
#28137=CARTESIAN_POINT('Origin',(8.75,-0.15,11.3));
#28138=CARTESIAN_POINT('Origin',(8.69,-0.7,10.79));
#28139=CARTESIAN_POINT('',(8.7,-0.7,10.79));
#28140=CARTESIAN_POINT('',(8.7,-0.1,10.79));
#28141=CARTESIAN_POINT('',(8.7,0.05,10.79));
#28142=CARTESIAN_POINT('',(8.75,-0.7,10.79));
#28143=CARTESIAN_POINT('',(8.69,-0.7,10.79));
#28144=CARTESIAN_POINT('',(8.75,-0.1,10.79));
#28145=CARTESIAN_POINT('',(8.75,-0.7,10.79));
#28146=CARTESIAN_POINT('',(8.69,-0.1,10.79));
#28147=CARTESIAN_POINT('Origin',(8.69,-0.1,10.79));
#28148=CARTESIAN_POINT('',(8.7,-0.1,10.81));
#28149=CARTESIAN_POINT('',(8.7,-0.1,6.395));
#28150=CARTESIAN_POINT('',(8.75,-0.1,10.81));
#28151=CARTESIAN_POINT('',(8.75,-0.1,10.79));
#28152=CARTESIAN_POINT('',(8.69,-0.1,10.81));
#28153=CARTESIAN_POINT('Origin',(8.69,-0.1,10.81));
#28154=CARTESIAN_POINT('',(8.7,-0.7,10.81));
#28155=CARTESIAN_POINT('',(8.7,0.35,10.81));
#28156=CARTESIAN_POINT('',(8.75,-0.7,10.81));
#28157=CARTESIAN_POINT('',(8.75,-0.1,10.81));
#28158=CARTESIAN_POINT('',(8.69,-0.7,10.81));
#28159=CARTESIAN_POINT('Origin',(8.69,-0.7,10.81));
#28160=CARTESIAN_POINT('',(8.7,-0.7,6.405));
#28161=CARTESIAN_POINT('',(8.75,-0.7,10.81));
#28162=CARTESIAN_POINT('Origin',(8.75,-0.4,10.8));
#28163=CARTESIAN_POINT('Origin',(8.69,-0.7,10.29));
#28164=CARTESIAN_POINT('',(8.7,-0.7,10.29));
#28165=CARTESIAN_POINT('',(8.7,0.4,10.29));
#28166=CARTESIAN_POINT('',(8.7,0.05,10.29));
#28167=CARTESIAN_POINT('',(8.75,-0.7,10.29));
#28168=CARTESIAN_POINT('',(8.69,-0.7,10.29));
#28169=CARTESIAN_POINT('',(8.75,0.4,10.29));
#28170=CARTESIAN_POINT('',(8.75,-0.7,10.29));
#28171=CARTESIAN_POINT('',(8.69,0.4,10.29));
#28172=CARTESIAN_POINT('Origin',(8.69,0.4,10.29));
#28173=CARTESIAN_POINT('',(8.7,0.4,10.31));
#28174=CARTESIAN_POINT('',(8.7,0.4,6.145));
#28175=CARTESIAN_POINT('',(8.75,0.4,10.31));
#28176=CARTESIAN_POINT('',(8.75,0.4,10.29));
#28177=CARTESIAN_POINT('',(8.69,0.4,10.31));
#28178=CARTESIAN_POINT('Origin',(8.69,0.4,10.31));
#28179=CARTESIAN_POINT('',(8.7,-0.7,10.31));
#28180=CARTESIAN_POINT('',(8.7,0.6,10.31));
#28181=CARTESIAN_POINT('',(8.75,-0.7,10.31));
#28182=CARTESIAN_POINT('',(8.75,0.4,10.31));
#28183=CARTESIAN_POINT('',(8.69,-0.7,10.31));
#28184=CARTESIAN_POINT('Origin',(8.69,-0.7,10.31));
#28185=CARTESIAN_POINT('',(8.7,-0.7,6.155));
#28186=CARTESIAN_POINT('',(8.75,-0.7,10.31));
#28187=CARTESIAN_POINT('Origin',(8.75,-0.15,10.3));
#28188=CARTESIAN_POINT('Origin',(8.69,-0.7,9.79));
#28189=CARTESIAN_POINT('',(8.7,-0.7,9.79));
#28190=CARTESIAN_POINT('',(8.7,-0.1,9.79));
#28191=CARTESIAN_POINT('',(8.7,0.05,9.79));
#28192=CARTESIAN_POINT('',(8.75,-0.7,9.79));
#28193=CARTESIAN_POINT('',(8.69,-0.7,9.79));
#28194=CARTESIAN_POINT('',(8.75,-0.1,9.79));
#28195=CARTESIAN_POINT('',(8.75,-0.7,9.79));
#28196=CARTESIAN_POINT('',(8.69,-0.1,9.79));
#28197=CARTESIAN_POINT('Origin',(8.69,-0.1,9.79));
#28198=CARTESIAN_POINT('',(8.7,-0.1,9.81));
#28199=CARTESIAN_POINT('',(8.7,-0.1,5.895));
#28200=CARTESIAN_POINT('',(8.75,-0.1,9.81));
#28201=CARTESIAN_POINT('',(8.75,-0.1,9.79));
#28202=CARTESIAN_POINT('',(8.69,-0.1,9.81));
#28203=CARTESIAN_POINT('Origin',(8.69,-0.1,9.81));
#28204=CARTESIAN_POINT('',(8.7,-0.7,9.81));
#28205=CARTESIAN_POINT('',(8.7,0.35,9.81));
#28206=CARTESIAN_POINT('',(8.75,-0.7,9.81));
#28207=CARTESIAN_POINT('',(8.75,-0.1,9.81));
#28208=CARTESIAN_POINT('',(8.69,-0.7,9.81));
#28209=CARTESIAN_POINT('Origin',(8.69,-0.7,9.81));
#28210=CARTESIAN_POINT('',(8.7,-0.7,5.905));
#28211=CARTESIAN_POINT('',(8.75,-0.7,9.81));
#28212=CARTESIAN_POINT('Origin',(8.75,-0.4,9.8));
#28213=CARTESIAN_POINT('Origin',(8.69,-0.7,9.29));
#28214=CARTESIAN_POINT('',(8.7,-0.7,9.29));
#28215=CARTESIAN_POINT('',(8.7,0.4,9.29));
#28216=CARTESIAN_POINT('',(8.7,0.05,9.29));
#28217=CARTESIAN_POINT('',(8.75,-0.7,9.29));
#28218=CARTESIAN_POINT('',(8.69,-0.7,9.29));
#28219=CARTESIAN_POINT('',(8.75,0.4,9.29));
#28220=CARTESIAN_POINT('',(8.75,-0.7,9.29));
#28221=CARTESIAN_POINT('',(8.69,0.4,9.29));
#28222=CARTESIAN_POINT('Origin',(8.69,0.4,9.29));
#28223=CARTESIAN_POINT('',(8.7,0.4,9.31));
#28224=CARTESIAN_POINT('',(8.7,0.4,5.645));
#28225=CARTESIAN_POINT('',(8.75,0.4,9.31));
#28226=CARTESIAN_POINT('',(8.75,0.4,9.29));
#28227=CARTESIAN_POINT('',(8.69,0.4,9.31));
#28228=CARTESIAN_POINT('Origin',(8.69,0.4,9.31));
#28229=CARTESIAN_POINT('',(8.7,-0.7,9.31));
#28230=CARTESIAN_POINT('',(8.7,0.6,9.31));
#28231=CARTESIAN_POINT('',(8.75,-0.7,9.31));
#28232=CARTESIAN_POINT('',(8.75,0.4,9.31));
#28233=CARTESIAN_POINT('',(8.69,-0.7,9.31));
#28234=CARTESIAN_POINT('Origin',(8.69,-0.7,9.31));
#28235=CARTESIAN_POINT('',(8.7,-0.7,5.655));
#28236=CARTESIAN_POINT('',(8.75,-0.7,9.31));
#28237=CARTESIAN_POINT('Origin',(8.75,-0.15,9.3));
#28238=CARTESIAN_POINT('Origin',(8.6,0.,28.));
#28239=CARTESIAN_POINT('',(8.7,-3.3677786976552E-17,28.275));
#28240=CARTESIAN_POINT('Origin',(8.7,0.,28.));
#28241=CARTESIAN_POINT('',(9.,3.3677786976552E-17,28.275));
#28242=CARTESIAN_POINT('',(8.6,-3.3677786976552E-17,28.275));
#28243=CARTESIAN_POINT('Origin',(9.,0.,28.));
#28244=CARTESIAN_POINT('Origin',(8.6,0.,3.));
#28245=CARTESIAN_POINT('',(8.7,-3.36777869765522E-17,3.275));
#28246=CARTESIAN_POINT('Origin',(8.7,0.,3.));
#28247=CARTESIAN_POINT('',(9.,3.36777869765522E-17,3.275));
#28248=CARTESIAN_POINT('',(8.6,-3.36777869765522E-17,3.275));
#28249=CARTESIAN_POINT('Origin',(9.,0.,3.));
#28250=CARTESIAN_POINT('Origin',(9.,0.8,2.));
#28251=CARTESIAN_POINT('',(9.,0.8,2.));
#28252=CARTESIAN_POINT('',(8.7,0.8,2.));
#28253=CARTESIAN_POINT('',(9.,0.8,2.));
#28254=CARTESIAN_POINT('',(8.7,0.8,30.));
#28255=CARTESIAN_POINT('',(8.7,0.8,2.));
#28256=CARTESIAN_POINT('',(9.,0.8,30.));
#28257=CARTESIAN_POINT('',(9.,0.8,30.));
#28258=CARTESIAN_POINT('',(9.,0.8,2.));
#28259=CARTESIAN_POINT('Origin',(9.,-0.8,2.));
#28260=CARTESIAN_POINT('',(9.,-0.8,2.));
#28261=CARTESIAN_POINT('',(9.,-0.8,2.));
#28262=CARTESIAN_POINT('',(9.,-0.8,30.));
#28263=CARTESIAN_POINT('',(9.,-0.8,30.));
#28264=CARTESIAN_POINT('',(9.,-0.8,2.));
#28265=CARTESIAN_POINT('Origin',(8.7,-0.8,2.));
#28266=CARTESIAN_POINT('',(8.7,-0.8,2.));
#28267=CARTESIAN_POINT('',(8.7,-0.8,2.));
#28268=CARTESIAN_POINT('',(8.7,-0.8,30.));
#28269=CARTESIAN_POINT('',(8.7,-0.8,30.));
#28270=CARTESIAN_POINT('',(8.7,-0.8,2.));
#28271=CARTESIAN_POINT('Origin',(8.7,0.8,2.));
#28272=CARTESIAN_POINT('',(8.7,0.8,2.));
#28273=CARTESIAN_POINT('',(8.7,0.8,30.));
#28274=CARTESIAN_POINT('Origin',(8.85,0.,30.));
#28275=CARTESIAN_POINT('Origin',(8.85,0.,2.));
#43407=UNCERTAINTY_MEASURE_WITH_UNIT(LENGTH_MEASURE(0.001),#43522,
'DISTANCE_ACCURACY_VALUE',
'Maximum model space distance between geometric entities at asserted c
onnectivities');
#43453=UNCERTAINTY_MEASURE_WITH_UNIT(LENGTH_MEASURE(0.001),#43522,
'DISTANCE_ACCURACY_VALUE',
'Maximum model space distance between geometric entities at asserted c
onnectivities');
#43475=(
GEOMETRIC_REPRESENTATION_CONTEXT(3)
GLOBAL_UNCERTAINTY_ASSIGNED_CONTEXT((#43407))
GLOBAL_UNIT_ASSIGNED_CONTEXT((#43522,#43524,#43525))
REPRESENTATION_CONTEXT('','3D')
);
#43521=(
GEOMETRIC_REPRESENTATION_CONTEXT(3)
GLOBAL_UNCERTAINTY_ASSIGNED_CONTEXT((#43453))
GLOBAL_UNIT_ASSIGNED_CONTEXT((#43522,#43524,#43525))
REPRESENTATION_CONTEXT('','3D')
);
#43522=(
LENGTH_UNIT()
NAMED_UNIT(*)
SI_UNIT(.CENTI.,.METRE.)
);
#43524=(
NAMED_UNIT(*)
PLANE_ANGLE_UNIT()
SI_UNIT($,.RADIAN.)
);
#43525=(
NAMED_UNIT(*)
SI_UNIT($,.STERADIAN.)
SOLID_ANGLE_UNIT()
);
#43547=SHAPE_DEFINITION_REPRESENTATION(#43614,#43815);
#43614=PRODUCT_DEFINITION_SHAPE('',$,#43883);
#43815=SHAPE_REPRESENTATION('',(#19782),#43475);
#43861=PRODUCT_DEFINITION_CONTEXT('part definition',#44064,'design');
#43883=PRODUCT_DEFINITION('Graduated scale','Graduated scale',#43950,#43861);
#43950=PRODUCT_DEFINITION_FORMATION('',$,#44087);
#44064=APPLICATION_CONTEXT(
'Core Data for Automotive Mechanical Design Process');
#44065=PRODUCT_CONTEXT('part definition',#44064,'mechanical');
#44087=PRODUCT('Graduated scale','Graduated scale','Graduated scale',(#44065));
#44210=COLOUR_RGB('Off White',0.89,0.88,0.83);
#44211=FILL_AREA_STYLE_COLOUR('',#44210);
#44212=FILL_AREA_STYLE('',(#44211));
#44213=SURFACE_STYLE_FILL_AREA(#44212);
#44214=SURFACE_SIDE_STYLE('',(#44213));
#44215=SURFACE_STYLE_USAGE(.BOTH.,#44214);
#44216=PRESENTATION_STYLE_ASSIGNMENT((#44215));
ENDSEC;
END-ISO-10303-21;
